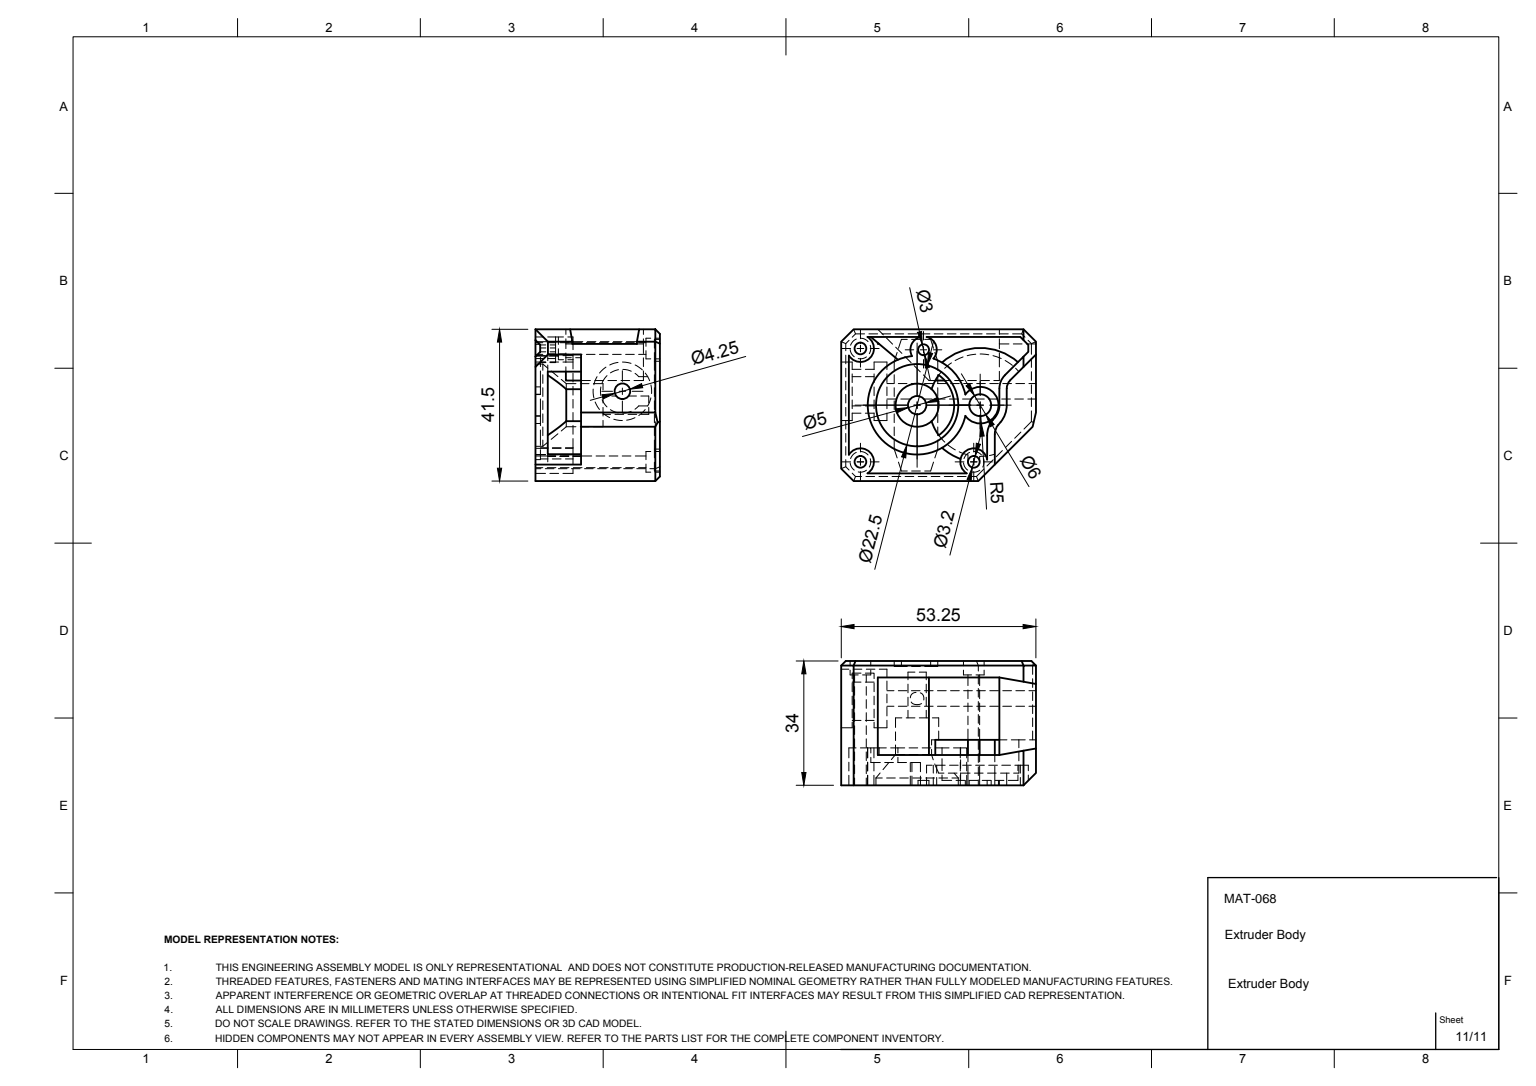
ISO-10303-21;
HEADER;
/* Generated by software containing ST-Developer
 * from STEP Tools, Inc. (www.steptools.com) 
 */

FILE_DESCRIPTION(
/* description */ ('CAx-IF Rec.Pracs.---Representation and Presentation of Product Manufa
cturing Information (PMI)---4.0---2014-10-13'),
/* implementation_level */ '2;1');

FILE_NAME(
/* name */ 'Extruder Body.step',
/* time_stamp */ '2026-10-24T16:53:48-07:00',
/* author */ (''),
/* organization */ (''),
/* preprocessor_version */ 'ST-DEVELOPER v20.2',
/* originating_system */ 'Autodesk Translation Framework v15.17.0.0',
/* authorisation */ '');

FILE_SCHEMA (('AP242_MANAGED_MODEL_BASED_3D_ENGINEERING_MIM_LF { 1 0 10303 442 2 1 4 }'));
ENDSEC;

DATA;
#10=MECHANICAL_DESIGN_GEOMETRIC_PRESENTATION_REPRESENTATION('',(#3498),#107910);
#883=CONICAL_SURFACE('',#50193,0.005875,0.694738276196703);
#2195=B_SPLINE_CURVE_WITH_KNOTS('',3,(#107237,#107238,#107239,#107240,#107241,
#107242,#107243,#107244,#107245,#107246,#107247,#107248,#107249,#107250,
#107251,#107252,#107253,#107254,#107255,#107256,#107257,#107258,#107259,
#107260,#107261,#107262,#107263,#107264,#107265,#107266,#107267,#107268,
#107269,#107270,#107271,#107272,#107273,#107274,#107275,#107276,#107277,
#107278),.UNSPECIFIED.,.T.,.F.,(4,2,2,2,2,2,2,2,2,2,2,2,2,2,2,2,2,2,2,2,
4),(0.,0.0683756752227249,0.13675135044545,0.193430456509981,0.239974549812452,
0.286518643114923,0.333062736417395,0.379606829719866,0.436285935784398,
0.504661611007122,0.573037286229846,0.641412961452571,0.709788636675295,
0.766467742739827,0.813011836042298,0.859555929344769,0.906100022647241,
0.952644115949712,1.00932322201424,1.07769889723697,1.14607457245969),
 .UNSPECIFIED.);
#2196=B_SPLINE_CURVE_WITH_KNOTS('',3,(#107310,#107311,#107312,#107313,#107314,
#107315,#107316,#107317),.UNSPECIFIED.,.F.,.F.,(4,2,2,4),(3.52079202383874,
3.52667424117723,4.17784077952384,4.18520413953086),.UNSPECIFIED.);
#2197=B_SPLINE_CURVE_WITH_KNOTS('',3,(#107322,#107323,#107324,#107325,#107326,
#107327,#107328,#107329),.UNSPECIFIED.,.F.,.F.,(4,2,2,4),(1.56581126613039,
1.57317462613742,2.22434116448402,2.23022338182252),.UNSPECIFIED.);
#3478=SHAPE_REPRESENTATION_RELATIONSHIP('SRR','None',#107956,#3488);
#3488=ADVANCED_BREP_SHAPE_REPRESENTATION('',(#3508),#107909);
#3498=STYLED_ITEM('',(#108007),#3508);
#3508=MANIFOLD_SOLID_BREP('Body1',#45546);
#3523=FACE_BOUND('',#9512,.T.);
#3524=FACE_BOUND('',#9516,.T.);
#3525=FACE_BOUND('',#9542,.T.);
#3526=FACE_BOUND('',#9543,.T.);
#3527=FACE_BOUND('',#9544,.T.);
#3528=FACE_BOUND('',#9545,.T.);
#3529=FACE_BOUND('',#9547,.T.);
#3530=FACE_BOUND('',#9548,.T.);
#3531=FACE_BOUND('',#9549,.T.);
#3532=FACE_BOUND('',#9550,.T.);
#3533=FACE_BOUND('',#9551,.T.);
#3534=FACE_BOUND('',#9552,.T.);
#3535=FACE_BOUND('',#9557,.T.);
#3536=FACE_BOUND('',#9563,.T.);
#3537=FACE_BOUND('',#9573,.T.);
#3538=FACE_BOUND('',#9575,.T.);
#3539=FACE_BOUND('',#9577,.T.);
#3540=FACE_BOUND('',#9607,.T.);
#3541=FACE_BOUND('',#9633,.T.);
#3682=PLANE('',#50239);
#3683=PLANE('',#50245);
#3684=PLANE('',#50248);
#3685=PLANE('',#50249);
#3686=PLANE('',#50250);
#3687=PLANE('',#50251);
#3688=PLANE('',#50263);
#3689=PLANE('',#50264);
#3690=PLANE('',#50265);
#3691=PLANE('',#50266);
#3692=PLANE('',#50276);
#3693=PLANE('',#50277);
#3694=PLANE('',#50278);
#3695=PLANE('',#50279);
#3696=PLANE('',#50280);
#3697=PLANE('',#50281);
#3698=PLANE('',#50282);
#3699=PLANE('',#50283);
#3700=PLANE('',#50284);
#3701=PLANE('',#50285);
#3702=PLANE('',#50286);
#3703=PLANE('',#50287);
#3704=PLANE('',#50288);
#3705=PLANE('',#50289);
#3706=PLANE('',#50290);
#3707=PLANE('',#50291);
#3708=PLANE('',#50292);
#3709=PLANE('',#50293);
#3710=PLANE('',#50294);
#3711=PLANE('',#50295);
#3712=PLANE('',#50296);
#3713=PLANE('',#50299);
#3714=PLANE('',#50302);
#3715=PLANE('',#50305);
#3716=PLANE('',#50308);
#3717=PLANE('',#50309);
#3718=PLANE('',#50310);
#3719=PLANE('',#50311);
#3720=PLANE('',#50314);
#3721=PLANE('',#50317);
#3722=PLANE('',#50318);
#3723=PLANE('',#50319);
#3724=PLANE('',#50321);
#3725=PLANE('',#50323);
#3726=PLANE('',#50325);
#3727=PLANE('',#50326);
#3728=PLANE('',#50329);
#3729=PLANE('',#50330);
#3730=PLANE('',#50331);
#3731=PLANE('',#50332);
#3732=PLANE('',#50333);
#3733=PLANE('',#50334);
#3734=PLANE('',#50335);
#3735=PLANE('',#50336);
#3736=PLANE('',#50337);
#3737=PLANE('',#50338);
#3738=PLANE('',#50339);
#3739=PLANE('',#50340);
#3740=PLANE('',#50341);
#3741=PLANE('',#50342);
#3742=PLANE('',#50345);
#3743=PLANE('',#50346);
#3744=PLANE('',#50349);
#3745=PLANE('',#50350);
#3746=PLANE('',#50351);
#3747=PLANE('',#50352);
#3748=PLANE('',#50353);
#3749=PLANE('',#50354);
#3750=PLANE('',#50355);
#3751=PLANE('',#50356);
#3752=PLANE('',#50357);
#3753=PLANE('',#50358);
#3754=PLANE('',#50359);
#3755=PLANE('',#50363);
#3756=PLANE('',#50364);
#3757=PLANE('',#50365);
#6572=FACE_OUTER_BOUND('',#9510,.T.);
#6573=FACE_OUTER_BOUND('',#9511,.T.);
#6574=FACE_OUTER_BOUND('',#9513,.T.);
#6575=FACE_OUTER_BOUND('',#9514,.T.);
#6576=FACE_OUTER_BOUND('',#9515,.T.);
#6577=FACE_OUTER_BOUND('',#9517,.T.);
#6578=FACE_OUTER_BOUND('',#9518,.T.);
#6579=FACE_OUTER_BOUND('',#9519,.T.);
#6580=FACE_OUTER_BOUND('',#9520,.T.);
#6581=FACE_OUTER_BOUND('',#9521,.T.);
#6582=FACE_OUTER_BOUND('',#9522,.T.);
#6583=FACE_OUTER_BOUND('',#9523,.T.);
#6584=FACE_OUTER_BOUND('',#9524,.T.);
#6585=FACE_OUTER_BOUND('',#9525,.T.);
#6586=FACE_OUTER_BOUND('',#9526,.T.);
#6587=FACE_OUTER_BOUND('',#9527,.T.);
#6588=FACE_OUTER_BOUND('',#9528,.T.);
#6589=FACE_OUTER_BOUND('',#9529,.T.);
#6590=FACE_OUTER_BOUND('',#9530,.T.);
#6591=FACE_OUTER_BOUND('',#9531,.T.);
#6592=FACE_OUTER_BOUND('',#9532,.T.);
#6593=FACE_OUTER_BOUND('',#9533,.T.);
#6594=FACE_OUTER_BOUND('',#9534,.T.);
#6595=FACE_OUTER_BOUND('',#9535,.T.);
#6596=FACE_OUTER_BOUND('',#9536,.T.);
#6597=FACE_OUTER_BOUND('',#9537,.T.);
#6598=FACE_OUTER_BOUND('',#9538,.T.);
#6599=FACE_OUTER_BOUND('',#9539,.T.);
#6600=FACE_OUTER_BOUND('',#9540,.T.);
#6601=FACE_OUTER_BOUND('',#9541,.T.);
#6602=FACE_OUTER_BOUND('',#9546,.T.);
#6603=FACE_OUTER_BOUND('',#9553,.T.);
#6604=FACE_OUTER_BOUND('',#9554,.T.);
#6605=FACE_OUTER_BOUND('',#9555,.T.);
#6606=FACE_OUTER_BOUND('',#9556,.T.);
#6607=FACE_OUTER_BOUND('',#9558,.T.);
#6608=FACE_OUTER_BOUND('',#9559,.T.);
#6609=FACE_OUTER_BOUND('',#9560,.T.);
#6610=FACE_OUTER_BOUND('',#9561,.T.);
#6611=FACE_OUTER_BOUND('',#9562,.T.);
#6612=FACE_OUTER_BOUND('',#9564,.T.);
#6613=FACE_OUTER_BOUND('',#9565,.T.);
#6614=FACE_OUTER_BOUND('',#9566,.T.);
#6615=FACE_OUTER_BOUND('',#9567,.T.);
#6616=FACE_OUTER_BOUND('',#9568,.T.);
#6617=FACE_OUTER_BOUND('',#9569,.T.);
#6618=FACE_OUTER_BOUND('',#9570,.T.);
#6619=FACE_OUTER_BOUND('',#9571,.T.);
#6620=FACE_OUTER_BOUND('',#9572,.T.);
#6621=FACE_OUTER_BOUND('',#9574,.T.);
#6622=FACE_OUTER_BOUND('',#9576,.T.);
#6623=FACE_OUTER_BOUND('',#9578,.T.);
#6624=FACE_OUTER_BOUND('',#9579,.T.);
#6625=FACE_OUTER_BOUND('',#9580,.T.);
#6626=FACE_OUTER_BOUND('',#9581,.T.);
#6627=FACE_OUTER_BOUND('',#9582,.T.);
#6628=FACE_OUTER_BOUND('',#9583,.T.);
#6629=FACE_OUTER_BOUND('',#9584,.T.);
#6630=FACE_OUTER_BOUND('',#9585,.T.);
#6631=FACE_OUTER_BOUND('',#9586,.T.);
#6632=FACE_OUTER_BOUND('',#9587,.T.);
#6633=FACE_OUTER_BOUND('',#9588,.T.);
#6634=FACE_OUTER_BOUND('',#9589,.T.);
#6635=FACE_OUTER_BOUND('',#9590,.T.);
#6636=FACE_OUTER_BOUND('',#9591,.T.);
#6637=FACE_OUTER_BOUND('',#9592,.T.);
#6638=FACE_OUTER_BOUND('',#9593,.T.);
#6639=FACE_OUTER_BOUND('',#9594,.T.);
#6640=FACE_OUTER_BOUND('',#9595,.T.);
#6641=FACE_OUTER_BOUND('',#9596,.T.);
#6642=FACE_OUTER_BOUND('',#9597,.T.);
#6643=FACE_OUTER_BOUND('',#9598,.T.);
#6644=FACE_OUTER_BOUND('',#9599,.T.);
#6645=FACE_OUTER_BOUND('',#9600,.T.);
#6646=FACE_OUTER_BOUND('',#9601,.T.);
#6647=FACE_OUTER_BOUND('',#9602,.T.);
#6648=FACE_OUTER_BOUND('',#9603,.T.);
#6649=FACE_OUTER_BOUND('',#9604,.T.);
#6650=FACE_OUTER_BOUND('',#9605,.T.);
#6651=FACE_OUTER_BOUND('',#9606,.T.);
#6652=FACE_OUTER_BOUND('',#9608,.T.);
#6653=FACE_OUTER_BOUND('',#9609,.T.);
#6654=FACE_OUTER_BOUND('',#9610,.T.);
#6655=FACE_OUTER_BOUND('',#9611,.T.);
#6656=FACE_OUTER_BOUND('',#9612,.T.);
#6657=FACE_OUTER_BOUND('',#9613,.T.);
#6658=FACE_OUTER_BOUND('',#9614,.T.);
#6659=FACE_OUTER_BOUND('',#9615,.T.);
#6660=FACE_OUTER_BOUND('',#9616,.T.);
#6661=FACE_OUTER_BOUND('',#9617,.T.);
#6662=FACE_OUTER_BOUND('',#9618,.T.);
#6663=FACE_OUTER_BOUND('',#9619,.T.);
#6664=FACE_OUTER_BOUND('',#9620,.T.);
#6665=FACE_OUTER_BOUND('',#9621,.T.);
#6666=FACE_OUTER_BOUND('',#9622,.T.);
#6667=FACE_OUTER_BOUND('',#9623,.T.);
#6668=FACE_OUTER_BOUND('',#9624,.T.);
#6669=FACE_OUTER_BOUND('',#9625,.T.);
#6670=FACE_OUTER_BOUND('',#9626,.T.);
#6671=FACE_OUTER_BOUND('',#9627,.T.);
#6672=FACE_OUTER_BOUND('',#9628,.T.);
#6673=FACE_OUTER_BOUND('',#9629,.T.);
#6674=FACE_OUTER_BOUND('',#9630,.T.);
#6675=FACE_OUTER_BOUND('',#9631,.T.);
#6676=FACE_OUTER_BOUND('',#9632,.T.);
#6677=FACE_OUTER_BOUND('',#9634,.T.);
#6678=FACE_OUTER_BOUND('',#9635,.T.);
#6679=FACE_OUTER_BOUND('',#9636,.T.);
#6680=FACE_OUTER_BOUND('',#9637,.T.);
#6681=FACE_OUTER_BOUND('',#9638,.T.);
#9510=EDGE_LOOP('',(#41354,#41355,#41356,#41357,#41358,#41359,#41360,#41361,
#41362,#41363,#41364,#41365));
#9511=EDGE_LOOP('',(#41366,#41367,#41368,#41369));
#9512=EDGE_LOOP('',(#41370));
#9513=EDGE_LOOP('',(#41371,#41372,#41373,#41374));
#9514=EDGE_LOOP('',(#41375,#41376,#41377,#41378));
#9515=EDGE_LOOP('',(#41379,#41380,#41381,#41382));
#9516=EDGE_LOOP('',(#41383));
#9517=EDGE_LOOP('',(#41384,#41385,#41386,#41387,#41388,#41389,#41390,#41391,
#41392));
#9518=EDGE_LOOP('',(#41393,#41394,#41395,#41396));
#9519=EDGE_LOOP('',(#41397,#41398,#41399,#41400));
#9520=EDGE_LOOP('',(#41401,#41402,#41403,#41404));
#9521=EDGE_LOOP('',(#41405,#41406,#41407,#41408,#41409,#41410));
#9522=EDGE_LOOP('',(#41411,#41412,#41413,#41414));
#9523=EDGE_LOOP('',(#41415,#41416,#41417,#41418));
#9524=EDGE_LOOP('',(#41419,#41420,#41421,#41422));
#9525=EDGE_LOOP('',(#41423,#41424,#41425,#41426));
#9526=EDGE_LOOP('',(#41427,#41428,#41429,#41430,#41431,#41432,#41433,#41434,
#41435,#41436));
#9527=EDGE_LOOP('',(#41437,#41438,#41439,#41440));
#9528=EDGE_LOOP('',(#41441,#41442,#41443,#41444,#41445,#41446,#41447,#41448));
#9529=EDGE_LOOP('',(#41449,#41450,#41451,#41452,#41453,#41454,#41455,#41456));
#9530=EDGE_LOOP('',(#41457,#41458,#41459,#41460));
#9531=EDGE_LOOP('',(#41461,#41462,#41463,#41464,#41465,#41466,#41467,#41468,
#41469));
#9532=EDGE_LOOP('',(#41470,#41471,#41472,#41473,#41474,#41475,#41476,#41477,
#41478,#41479,#41480,#41481,#41482,#41483,#41484));
#9533=EDGE_LOOP('',(#41485,#41486,#41487,#41488,#41489,#41490));
#9534=EDGE_LOOP('',(#41491,#41492,#41493,#41494,#41495));
#9535=EDGE_LOOP('',(#41496,#41497,#41498,#41499));
#9536=EDGE_LOOP('',(#41500,#41501,#41502,#41503,#41504,#41505,#41506,#41507,
#41508,#41509,#41510,#41511,#41512));
#9537=EDGE_LOOP('',(#41513,#41514,#41515,#41516,#41517,#41518));
#9538=EDGE_LOOP('',(#41519,#41520,#41521,#41522,#41523));
#9539=EDGE_LOOP('',(#41524,#41525,#41526,#41527));
#9540=EDGE_LOOP('',(#41528,#41529,#41530,#41531,#41532,#41533));
#9541=EDGE_LOOP('',(#41534,#41535,#41536,#41537,#41538,#41539,#41540,#41541));
#9542=EDGE_LOOP('',(#41542,#41543,#41544,#41545,#41546,#41547,#41548,#41549));
#9543=EDGE_LOOP('',(#41550));
#9544=EDGE_LOOP('',(#41551));
#9545=EDGE_LOOP('',(#41552));
#9546=EDGE_LOOP('',(#41553,#41554,#41555,#41556,#41557,#41558,#41559,#41560,
#41561,#41562,#41563,#41564,#41565,#41566,#41567,#41568,#41569,#41570,#41571,
#41572,#41573,#41574,#41575,#41576,#41577,#41578,#41579,#41580,#41581,#41582,
#41583,#41584,#41585,#41586,#41587));
#9547=EDGE_LOOP('',(#41588));
#9548=EDGE_LOOP('',(#41589));
#9549=EDGE_LOOP('',(#41590));
#9550=EDGE_LOOP('',(#41591));
#9551=EDGE_LOOP('',(#41592));
#9552=EDGE_LOOP('',(#41593));
#9553=EDGE_LOOP('',(#41594,#41595,#41596,#41597));
#9554=EDGE_LOOP('',(#41598,#41599,#41600,#41601,#41602,#41603,#41604,#41605,
#41606,#41607));
#9555=EDGE_LOOP('',(#41608,#41609,#41610,#41611));
#9556=EDGE_LOOP('',(#41612,#41613,#41614,#41615,#41616,#41617,#41618,#41619,
#41620,#41621));
#9557=EDGE_LOOP('',(#41622));
#9558=EDGE_LOOP('',(#41623,#41624,#41625,#41626,#41627));
#9559=EDGE_LOOP('',(#41628,#41629,#41630,#41631,#41632,#41633));
#9560=EDGE_LOOP('',(#41634,#41635,#41636,#41637));
#9561=EDGE_LOOP('',(#41638,#41639,#41640,#41641));
#9562=EDGE_LOOP('',(#41642,#41643,#41644,#41645));
#9563=EDGE_LOOP('',(#41646));
#9564=EDGE_LOOP('',(#41647,#41648,#41649,#41650));
#9565=EDGE_LOOP('',(#41651,#41652,#41653,#41654));
#9566=EDGE_LOOP('',(#41655,#41656,#41657,#41658));
#9567=EDGE_LOOP('',(#41659,#41660,#41661,#41662));
#9568=EDGE_LOOP('',(#41663,#41664,#41665,#41666));
#9569=EDGE_LOOP('',(#41667,#41668,#41669,#41670,#41671));
#9570=EDGE_LOOP('',(#41672,#41673,#41674,#41675));
#9571=EDGE_LOOP('',(#41676,#41677,#41678,#41679,#41680));
#9572=EDGE_LOOP('',(#41681));
#9573=EDGE_LOOP('',(#41682));
#9574=EDGE_LOOP('',(#41683));
#9575=EDGE_LOOP('',(#41684));
#9576=EDGE_LOOP('',(#41685));
#9577=EDGE_LOOP('',(#41686));
#9578=EDGE_LOOP('',(#41687,#41688,#41689,#41690,#41691,#41692,#41693));
#9579=EDGE_LOOP('',(#41694,#41695,#41696,#41697));
#9580=EDGE_LOOP('',(#41698,#41699,#41700,#41701));
#9581=EDGE_LOOP('',(#41702,#41703,#41704,#41705));
#9582=EDGE_LOOP('',(#41706,#41707,#41708,#41709));
#9583=EDGE_LOOP('',(#41710,#41711,#41712,#41713));
#9584=EDGE_LOOP('',(#41714,#41715,#41716,#41717,#41718,#41719));
#9585=EDGE_LOOP('',(#41720,#41721,#41722,#41723));
#9586=EDGE_LOOP('',(#41724,#41725,#41726,#41727,#41728,#41729,#41730,#41731,
#41732,#41733,#41734,#41735,#41736,#41737,#41738));
#9587=EDGE_LOOP('',(#41739,#41740,#41741,#41742));
#9588=EDGE_LOOP('',(#41743,#41744,#41745,#41746));
#9589=EDGE_LOOP('',(#41747,#41748,#41749,#41750));
#9590=EDGE_LOOP('',(#41751,#41752,#41753,#41754));
#9591=EDGE_LOOP('',(#41755,#41756,#41757,#41758));
#9592=EDGE_LOOP('',(#41759,#41760,#41761,#41762));
#9593=EDGE_LOOP('',(#41763,#41764,#41765,#41766,#41767));
#9594=EDGE_LOOP('',(#41768,#41769,#41770,#41771));
#9595=EDGE_LOOP('',(#41772,#41773,#41774,#41775,#41776,#41777,#41778));
#9596=EDGE_LOOP('',(#41779,#41780,#41781,#41782));
#9597=EDGE_LOOP('',(#41783,#41784,#41785,#41786));
#9598=EDGE_LOOP('',(#41787,#41788,#41789,#41790));
#9599=EDGE_LOOP('',(#41791,#41792,#41793,#41794));
#9600=EDGE_LOOP('',(#41795,#41796,#41797,#41798));
#9601=EDGE_LOOP('',(#41799,#41800,#41801,#41802));
#9602=EDGE_LOOP('',(#41803,#41804,#41805,#41806,#41807,#41808,#41809,#41810));
#9603=EDGE_LOOP('',(#41811,#41812,#41813,#41814));
#9604=EDGE_LOOP('',(#41815));
#9605=EDGE_LOOP('',(#41816,#41817,#41818,#41819));
#9606=EDGE_LOOP('',(#41820));
#9607=EDGE_LOOP('',(#41821));
#9608=EDGE_LOOP('',(#41822));
#9609=EDGE_LOOP('',(#41823));
#9610=EDGE_LOOP('',(#41824,#41825,#41826,#41827));
#9611=EDGE_LOOP('',(#41828,#41829,#41830,#41831));
#9612=EDGE_LOOP('',(#41832,#41833,#41834,#41835));
#9613=EDGE_LOOP('',(#41836,#41837,#41838,#41839));
#9614=EDGE_LOOP('',(#41840,#41841,#41842,#41843));
#9615=EDGE_LOOP('',(#41844,#41845,#41846,#41847));
#9616=EDGE_LOOP('',(#41848,#41849,#41850,#41851));
#9617=EDGE_LOOP('',(#41852,#41853,#41854,#41855));
#9618=EDGE_LOOP('',(#41856,#41857,#41858,#41859,#41860,#41861,#41862,#41863));
#9619=EDGE_LOOP('',(#41864,#41865,#41866,#41867));
#9620=EDGE_LOOP('',(#41868,#41869,#41870,#41871,#41872,#41873,#41874));
#9621=EDGE_LOOP('',(#41875,#41876,#41877,#41878,#41879,#41880,#41881,#41882));
#9622=EDGE_LOOP('',(#41883,#41884,#41885,#41886));
#9623=EDGE_LOOP('',(#41887,#41888,#41889,#41890,#41891,#41892,#41893,#41894,
#41895,#41896,#41897,#41898));
#9624=EDGE_LOOP('',(#41899,#41900,#41901,#41902,#41903));
#9625=EDGE_LOOP('',(#41904,#41905,#41906,#41907,#41908));
#9626=EDGE_LOOP('',(#41909,#41910,#41911,#41912));
#9627=EDGE_LOOP('',(#41913,#41914,#41915));
#9628=EDGE_LOOP('',(#41916,#41917,#41918,#41919));
#9629=EDGE_LOOP('',(#41920,#41921,#41922,#41923));
#9630=EDGE_LOOP('',(#41924,#41925,#41926,#41927,#41928,#41929));
#9631=EDGE_LOOP('',(#41930,#41931,#41932,#41933,#41934,#41935));
#9632=EDGE_LOOP('',(#41936));
#9633=EDGE_LOOP('',(#41937));
#9634=EDGE_LOOP('',(#41938,#41939,#41940,#41941,#41942));
#9635=EDGE_LOOP('',(#41943,#41944,#41945,#41946));
#9636=EDGE_LOOP('',(#41947,#41948,#41949,#41950,#41951));
#9637=EDGE_LOOP('',(#41952,#41953,#41954,#41955));
#9638=EDGE_LOOP('',(#41956,#41957,#41958,#41959));
#11405=LINE('',#107215,#13389);
#11406=LINE('',#107219,#13390);
#11407=LINE('',#107223,#13391);
#11408=LINE('',#107228,#13392);
#11409=LINE('',#107234,#13393);
#11410=LINE('',#107283,#13394);
#11411=LINE('',#107290,#13395);
#11412=LINE('',#107293,#13396);
#11413=LINE('',#107298,#13397);
#11414=LINE('',#107305,#13398);
#11415=LINE('',#107332,#13399);
#11416=LINE('',#107338,#13400);
#11417=LINE('',#107345,#13401);
#11418=LINE('',#107348,#13402);
#11419=LINE('',#107354,#13403);
#11420=LINE('',#107358,#13404);
#11421=LINE('',#107361,#13405);
#11422=LINE('',#107366,#13406);
#11423=LINE('',#107372,#13407);
#11424=LINE('',#107378,#13408);
#11425=LINE('',#107384,#13409);
#11426=LINE('',#107390,#13410);
#11427=LINE('',#107394,#13411);
#11428=LINE('',#107398,#13412);
#11429=LINE('',#107400,#13413);
#11430=LINE('',#107405,#13414);
#11431=LINE('',#107409,#13415);
#11432=LINE('',#107412,#13416);
#11433=LINE('',#107415,#13417);
#11434=LINE('',#107421,#13418);
#11435=LINE('',#107426,#13419);
#11436=LINE('',#107429,#13420);
#11437=LINE('',#107433,#13421);
#11438=LINE('',#107435,#13422);
#11439=LINE('',#107437,#13423);
#11440=LINE('',#107438,#13424);
#11441=LINE('',#107442,#13425);
#11442=LINE('',#107446,#13426);
#11443=LINE('',#107450,#13427);
#11444=LINE('',#107455,#13428);
#11445=LINE('',#107458,#13429);
#11446=LINE('',#107460,#13430);
#11447=LINE('',#107464,#13431);
#11448=LINE('',#107466,#13432);
#11449=LINE('',#107468,#13433);
#11450=LINE('',#107470,#13434);
#11451=LINE('',#107471,#13435);
#11452=LINE('',#107472,#13436);
#11453=LINE('',#107476,#13437);
#11454=LINE('',#107478,#13438);
#11455=LINE('',#107479,#13439);
#11456=LINE('',#107480,#13440);
#11457=LINE('',#107481,#13441);
#11458=LINE('',#107485,#13442);
#11459=LINE('',#107487,#13443);
#11460=LINE('',#107488,#13444);
#11461=LINE('',#107490,#13445);
#11462=LINE('',#107491,#13446);
#11463=LINE('',#107495,#13447);
#11464=LINE('',#107497,#13448);
#11465=LINE('',#107499,#13449);
#11466=LINE('',#107500,#13450);
#11467=LINE('',#107504,#13451);
#11468=LINE('',#107508,#13452);
#11469=LINE('',#107512,#13453);
#11470=LINE('',#107516,#13454);
#11471=LINE('',#107522,#13455);
#11472=LINE('',#107528,#13456);
#11473=LINE('',#107531,#13457);
#11474=LINE('',#107533,#13458);
#11475=LINE('',#107534,#13459);
#11476=LINE('',#107538,#13460);
#11477=LINE('',#107540,#13461);
#11478=LINE('',#107542,#13462);
#11479=LINE('',#107544,#13463);
#11480=LINE('',#107546,#13464);
#11481=LINE('',#107547,#13465);
#11482=LINE('',#107551,#13466);
#11483=LINE('',#107553,#13467);
#11484=LINE('',#107555,#13468);
#11485=LINE('',#107557,#13469);
#11486=LINE('',#107559,#13470);
#11487=LINE('',#107561,#13471);
#11488=LINE('',#107563,#13472);
#11489=LINE('',#107564,#13473);
#11490=LINE('',#107567,#13474);
#11491=LINE('',#107569,#13475);
#11492=LINE('',#107571,#13476);
#11493=LINE('',#107573,#13477);
#11494=LINE('',#107575,#13478);
#11495=LINE('',#107577,#13479);
#11496=LINE('',#107579,#13480);
#11497=LINE('',#107580,#13481);
#11498=LINE('',#107583,#13482);
#11499=LINE('',#107585,#13483);
#11500=LINE('',#107587,#13484);
#11501=LINE('',#107589,#13485);
#11502=LINE('',#107591,#13486);
#11503=LINE('',#107593,#13487);
#11504=LINE('',#107595,#13488);
#11505=LINE('',#107597,#13489);
#11506=LINE('',#107599,#13490);
#11507=LINE('',#107603,#13491);
#11508=LINE('',#107607,#13492);
#11509=LINE('',#107611,#13493);
#11510=LINE('',#107613,#13494);
#11511=LINE('',#107615,#13495);
#11512=LINE('',#107619,#13496);
#11513=LINE('',#107623,#13497);
#11514=LINE('',#107626,#13498);
#11515=LINE('',#107628,#13499);
#11516=LINE('',#107632,#13500);
#11517=LINE('',#107637,#13501);
#11518=LINE('',#107639,#13502);
#11519=LINE('',#107640,#13503);
#11520=LINE('',#107642,#13504);
#11521=LINE('',#107643,#13505);
#11522=LINE('',#107645,#13506);
#11523=LINE('',#107646,#13507);
#11524=LINE('',#107647,#13508);
#11525=LINE('',#107651,#13509);
#11526=LINE('',#107652,#13510);
#11527=LINE('',#107653,#13511);
#11528=LINE('',#107655,#13512);
#11529=LINE('',#107656,#13513);
#11530=LINE('',#107658,#13514);
#11531=LINE('',#107659,#13515);
#11532=LINE('',#107661,#13516);
#11533=LINE('',#107662,#13517);
#11534=LINE('',#107665,#13518);
#11535=LINE('',#107667,#13519);
#11536=LINE('',#107668,#13520);
#11537=LINE('',#107670,#13521);
#11538=LINE('',#107672,#13522);
#11539=LINE('',#107673,#13523);
#11540=LINE('',#107676,#13524);
#11541=LINE('',#107677,#13525);
#11542=LINE('',#107680,#13526);
#11543=LINE('',#107681,#13527);
#11544=LINE('',#107683,#13528);
#11545=LINE('',#107685,#13529);
#11546=LINE('',#107686,#13530);
#11547=LINE('',#107688,#13531);
#11548=LINE('',#107690,#13532);
#11549=LINE('',#107692,#13533);
#11550=LINE('',#107694,#13534);
#11551=LINE('',#107696,#13535);
#11552=LINE('',#107698,#13536);
#11553=LINE('',#107704,#13537);
#11554=LINE('',#107706,#13538);
#11555=LINE('',#107707,#13539);
#11556=LINE('',#107710,#13540);
#11557=LINE('',#107714,#13541);
#11558=LINE('',#107715,#13542);
#11559=LINE('',#107718,#13543);
#11560=LINE('',#107722,#13544);
#11561=LINE('',#107723,#13545);
#11562=LINE('',#107726,#13546);
#11563=LINE('',#107730,#13547);
#11564=LINE('',#107731,#13548);
#11565=LINE('',#107734,#13549);
#11566=LINE('',#107737,#13550);
#11567=LINE('',#107738,#13551);
#11568=LINE('',#107743,#13552);
#11569=LINE('',#107744,#13553);
#11570=LINE('',#107748,#13554);
#11571=LINE('',#107751,#13555);
#11572=LINE('',#107752,#13556);
#11573=LINE('',#107758,#13557);
#11574=LINE('',#107759,#13558);
#11575=LINE('',#107760,#13559);
#11576=LINE('',#107764,#13560);
#11577=LINE('',#107765,#13561);
#11578=LINE('',#107766,#13562);
#11579=LINE('',#107768,#13563);
#11580=LINE('',#107770,#13564);
#11581=LINE('',#107771,#13565);
#11582=LINE('',#107772,#13566);
#11583=LINE('',#107774,#13567);
#11584=LINE('',#107776,#13568);
#11585=LINE('',#107778,#13569);
#11586=LINE('',#107780,#13570);
#11587=LINE('',#107782,#13571);
#11588=LINE('',#107789,#13572);
#11589=LINE('',#107795,#13573);
#11590=LINE('',#107797,#13574);
#11591=LINE('',#107798,#13575);
#11592=LINE('',#107801,#13576);
#11593=LINE('',#107802,#13577);
#11594=LINE('',#107805,#13578);
#11595=LINE('',#107806,#13579);
#11596=LINE('',#107809,#13580);
#11597=LINE('',#107810,#13581);
#11598=LINE('',#107813,#13582);
#11599=LINE('',#107814,#13583);
#11600=LINE('',#107817,#13584);
#11601=LINE('',#107818,#13585);
#11602=LINE('',#107821,#13586);
#11603=LINE('',#107822,#13587);
#11604=LINE('',#107824,#13588);
#11605=LINE('',#107831,#13589);
#11606=LINE('',#107833,#13590);
#11607=LINE('',#107835,#13591);
#11608=LINE('',#107837,#13592);
#11609=LINE('',#107838,#13593);
#11610=LINE('',#107843,#13594);
#11611=LINE('',#107844,#13595);
#11612=LINE('',#107848,#13596);
#11613=LINE('',#107851,#13597);
#11614=LINE('',#107852,#13598);
#11615=LINE('',#107854,#13599);
#11616=LINE('',#107857,#13600);
#11617=LINE('',#107864,#13601);
#11618=LINE('',#107865,#13602);
#11619=LINE('',#107870,#13603);
#11620=LINE('',#107871,#13604);
#11621=LINE('',#107873,#13605);
#11622=LINE('',#107874,#13606);
#13389=VECTOR('',#61178,0.008);
#13390=VECTOR('',#61181,1.);
#13391=VECTOR('',#61184,0.008);
#13392=VECTOR('',#61189,1.);
#13393=VECTOR('',#61196,0.002125);
#13394=VECTOR('',#61203,0.003);
#13395=VECTOR('',#61210,1.);
#13396=VECTOR('',#61213,1.);
#13397=VECTOR('',#61218,0.0025);
#13398=VECTOR('',#61225,0.005875);
#13399=VECTOR('',#61236,0.01125);
#13400=VECTOR('',#61243,0.0015);
#13401=VECTOR('',#61250,1.);
#13402=VECTOR('',#61253,1.);
#13403=VECTOR('',#61258,1.);
#13404=VECTOR('',#61261,1.);
#13405=VECTOR('',#61264,1.);
#13406=VECTOR('',#61269,0.002825);
#13407=VECTOR('',#61276,0.002825);
#13408=VECTOR('',#61283,0.002825);
#13409=VECTOR('',#61290,0.0016);
#13410=VECTOR('',#61297,0.0016);
#13411=VECTOR('',#61300,1.);
#13412=VECTOR('',#61303,0.0016);
#13413=VECTOR('',#61306,1.);
#13414=VECTOR('',#61311,0.0016);
#13415=VECTOR('',#61316,0.0059);
#13416=VECTOR('',#61319,1.);
#13417=VECTOR('',#61322,1.);
#13418=VECTOR('',#61327,1.);
#13419=VECTOR('',#61332,1.);
#13420=VECTOR('',#61335,1.);
#13421=VECTOR('',#61338,1.);
#13422=VECTOR('',#61339,1.);
#13423=VECTOR('',#61340,1.);
#13424=VECTOR('',#61341,1.);
#13425=VECTOR('',#61344,1.);
#13426=VECTOR('',#61347,1.);
#13427=VECTOR('',#61350,1.);
#13428=VECTOR('',#61357,1.);
#13429=VECTOR('',#61360,1.);
#13430=VECTOR('',#61361,1.);
#13431=VECTOR('',#61364,1.);
#13432=VECTOR('',#61365,1.);
#13433=VECTOR('',#61366,1.);
#13434=VECTOR('',#61367,1.);
#13435=VECTOR('',#61368,1.);
#13436=VECTOR('',#61369,1.);
#13437=VECTOR('',#61372,1.);
#13438=VECTOR('',#61373,1.);
#13439=VECTOR('',#61374,1.);
#13440=VECTOR('',#61375,1.);
#13441=VECTOR('',#61376,1.);
#13442=VECTOR('',#61379,1.);
#13443=VECTOR('',#61380,1.);
#13444=VECTOR('',#61381,1.);
#13445=VECTOR('',#61382,1.);
#13446=VECTOR('',#61383,1.);
#13447=VECTOR('',#61386,1.);
#13448=VECTOR('',#61387,1.);
#13449=VECTOR('',#61388,1.);
#13450=VECTOR('',#61389,1.);
#13451=VECTOR('',#61394,1.);
#13452=VECTOR('',#61397,1.);
#13453=VECTOR('',#61400,1.);
#13454=VECTOR('',#61403,1.);
#13455=VECTOR('',#61410,1.);
#13456=VECTOR('',#61419,1.);
#13457=VECTOR('',#61422,1.);
#13458=VECTOR('',#61423,1.);
#13459=VECTOR('',#61424,1.);
#13460=VECTOR('',#61427,1.);
#13461=VECTOR('',#61428,1.);
#13462=VECTOR('',#61429,1.);
#13463=VECTOR('',#61430,1.);
#13464=VECTOR('',#61431,1.);
#13465=VECTOR('',#61432,1.);
#13466=VECTOR('',#61435,1.);
#13467=VECTOR('',#61436,1.);
#13468=VECTOR('',#61437,1.);
#13469=VECTOR('',#61438,1.);
#13470=VECTOR('',#61439,1.);
#13471=VECTOR('',#61440,1.);
#13472=VECTOR('',#61441,1.);
#13473=VECTOR('',#61442,1.);
#13474=VECTOR('',#61443,1.);
#13475=VECTOR('',#61444,1.);
#13476=VECTOR('',#61445,1.);
#13477=VECTOR('',#61446,1.);
#13478=VECTOR('',#61447,1.);
#13479=VECTOR('',#61448,1.);
#13480=VECTOR('',#61449,1.);
#13481=VECTOR('',#61450,1.);
#13482=VECTOR('',#61453,1.);
#13483=VECTOR('',#61454,1.);
#13484=VECTOR('',#61455,1.);
#13485=VECTOR('',#61456,1.);
#13486=VECTOR('',#61457,1.);
#13487=VECTOR('',#61458,1.);
#13488=VECTOR('',#61459,1.);
#13489=VECTOR('',#61460,1.);
#13490=VECTOR('',#61461,1.);
#13491=VECTOR('',#61464,1.);
#13492=VECTOR('',#61467,1.);
#13493=VECTOR('',#61470,1.);
#13494=VECTOR('',#61471,1.);
#13495=VECTOR('',#61472,1.);
#13496=VECTOR('',#61475,1.);
#13497=VECTOR('',#61478,1.);
#13498=VECTOR('',#61481,1.);
#13499=VECTOR('',#61482,1.);
#13500=VECTOR('',#61485,1.);
#13501=VECTOR('',#61492,1.);
#13502=VECTOR('',#61493,1.);
#13503=VECTOR('',#61494,1.);
#13504=VECTOR('',#61497,1.);
#13505=VECTOR('',#61498,1.);
#13506=VECTOR('',#61499,1.);
#13507=VECTOR('',#61500,1.);
#13508=VECTOR('',#61501,1.);
#13509=VECTOR('',#61504,1.);
#13510=VECTOR('',#61505,1.);
#13511=VECTOR('',#61506,1.);
#13512=VECTOR('',#61509,1.);
#13513=VECTOR('',#61510,1.);
#13514=VECTOR('',#61511,1.);
#13515=VECTOR('',#61512,1.);
#13516=VECTOR('',#61513,1.);
#13517=VECTOR('',#61514,1.);
#13518=VECTOR('',#61517,1.);
#13519=VECTOR('',#61518,1.);
#13520=VECTOR('',#61519,1.);
#13521=VECTOR('',#61522,1.);
#13522=VECTOR('',#61523,1.);
#13523=VECTOR('',#61524,1.);
#13524=VECTOR('',#61527,1.);
#13525=VECTOR('',#61528,1.);
#13526=VECTOR('',#61531,1.);
#13527=VECTOR('',#61532,1.);
#13528=VECTOR('',#61535,1.);
#13529=VECTOR('',#61538,1.);
#13530=VECTOR('',#61539,1.);
#13531=VECTOR('',#61542,1.);
#13532=VECTOR('',#61545,1.);
#13533=VECTOR('',#61548,1.);
#13534=VECTOR('',#61551,1.);
#13535=VECTOR('',#61554,1.);
#13536=VECTOR('',#61557,1.);
#13537=VECTOR('',#61568,1.);
#13538=VECTOR('',#61569,1.);
#13539=VECTOR('',#61570,1.);
#13540=VECTOR('',#61573,1.);
#13541=VECTOR('',#61578,1.);
#13542=VECTOR('',#61579,1.);
#13543=VECTOR('',#61582,1.);
#13544=VECTOR('',#61587,1.);
#13545=VECTOR('',#61588,1.);
#13546=VECTOR('',#61591,1.);
#13547=VECTOR('',#61596,1.);
#13548=VECTOR('',#61597,1.);
#13549=VECTOR('',#61600,1.);
#13550=VECTOR('',#61605,1.);
#13551=VECTOR('',#61606,1.);
#13552=VECTOR('',#61613,1.);
#13553=VECTOR('',#61614,1.);
#13554=VECTOR('',#61619,1.);
#13555=VECTOR('',#61622,1.);
#13556=VECTOR('',#61623,1.);
#13557=VECTOR('',#61630,1.);
#13558=VECTOR('',#61631,1.);
#13559=VECTOR('',#61632,1.);
#13560=VECTOR('',#61635,1.);
#13561=VECTOR('',#61636,1.);
#13562=VECTOR('',#61637,1.);
#13563=VECTOR('',#61640,1.);
#13564=VECTOR('',#61641,1.);
#13565=VECTOR('',#61642,1.);
#13566=VECTOR('',#61643,1.);
#13567=VECTOR('',#61646,1.);
#13568=VECTOR('',#61649,1.);
#13569=VECTOR('',#61652,1.);
#13570=VECTOR('',#61655,1.);
#13571=VECTOR('',#61658,1.);
#13572=VECTOR('',#61671,1.);
#13573=VECTOR('',#61680,1.);
#13574=VECTOR('',#61681,1.);
#13575=VECTOR('',#61682,1.);
#13576=VECTOR('',#61685,1.);
#13577=VECTOR('',#61686,1.);
#13578=VECTOR('',#61689,1.);
#13579=VECTOR('',#61690,1.);
#13580=VECTOR('',#61693,1.);
#13581=VECTOR('',#61694,1.);
#13582=VECTOR('',#61697,1.);
#13583=VECTOR('',#61698,1.);
#13584=VECTOR('',#61701,1.);
#13585=VECTOR('',#61702,1.);
#13586=VECTOR('',#61705,1.);
#13587=VECTOR('',#61706,1.);
#13588=VECTOR('',#61709,1.);
#13589=VECTOR('',#61720,1.);
#13590=VECTOR('',#61721,1.);
#13591=VECTOR('',#61722,1.);
#13592=VECTOR('',#61723,1.);
#13593=VECTOR('',#61724,1.);
#13594=VECTOR('',#61731,1.);
#13595=VECTOR('',#61732,1.);
#13596=VECTOR('',#61739,1.);
#13597=VECTOR('',#61742,1.);
#13598=VECTOR('',#61743,1.);
#13599=VECTOR('',#61746,1.);
#13600=VECTOR('',#61751,1.);
#13601=VECTOR('',#61760,1.);
#13602=VECTOR('',#61761,1.);
#13603=VECTOR('',#61766,1.);
#13604=VECTOR('',#61767,1.);
#13605=VECTOR('',#61770,1.);
#13606=VECTOR('',#61771,1.);
#17097=CIRCLE('',#50175,0.00800000000000999);
#17098=CIRCLE('',#50176,0.00800000000000999);
#17099=CIRCLE('',#50177,0.00800000000000999);
#17100=CIRCLE('',#50178,0.00800000000000999);
#17101=CIRCLE('',#50179,0.00800000000000999);
#17102=CIRCLE('',#50180,0.00800000000000999);
#17103=CIRCLE('',#50182,0.00212500000001);
#17104=CIRCLE('',#50183,0.00212500000001);
#17105=CIRCLE('',#50185,0.00300000000001);
#17106=CIRCLE('',#50186,0.00300000000001);
#17107=CIRCLE('',#50188,0.00500000000001);
#17108=CIRCLE('',#50189,0.00500000000001);
#17109=CIRCLE('',#50191,0.00250000000001);
#17110=CIRCLE('',#50192,0.00250000000001);
#17111=CIRCLE('',#50194,0.01012500000001);
#17112=CIRCLE('',#50195,0.01125000000001);
#17113=CIRCLE('',#50196,0.01012500000001);
#17114=CIRCLE('',#50197,0.00590000000001);
#17115=CIRCLE('',#50198,0.00590000000001);
#17116=CIRCLE('',#50200,0.01125000000001);
#17117=CIRCLE('',#50202,0.00150000000001);
#17118=CIRCLE('',#50203,0.00150000000001);
#17119=CIRCLE('',#50205,0.00360000000001);
#17120=CIRCLE('',#50206,0.00360000000001);
#17121=CIRCLE('',#50208,0.00370000000001);
#17122=CIRCLE('',#50209,0.00370000000001);
#17123=CIRCLE('',#50210,0.00370000000001);
#17124=CIRCLE('',#50212,0.00282500000001);
#17125=CIRCLE('',#50213,0.00282500000001);
#17126=CIRCLE('',#50215,0.00282500000001);
#17127=CIRCLE('',#50216,0.00282500000001);
#17128=CIRCLE('',#50218,0.00282500000001);
#17129=CIRCLE('',#50219,0.00282500000001);
#17130=CIRCLE('',#50221,0.00160000000001);
#17131=CIRCLE('',#50222,0.00160000000001);
#17132=CIRCLE('',#50224,0.00160000000001);
#17133=CIRCLE('',#50225,0.00160000000001);
#17134=CIRCLE('',#50226,0.00160000000001);
#17135=CIRCLE('',#50227,0.00160000000001);
#17136=CIRCLE('',#50229,0.00160000000001);
#17137=CIRCLE('',#50230,0.00160000000001);
#17138=CIRCLE('',#50232,0.00590000000001);
#17139=CIRCLE('',#50233,0.00590000000001);
#17140=CIRCLE('',#50235,0.01350000000001);
#17141=CIRCLE('',#50236,0.01350000000001);
#17142=CIRCLE('',#50237,0.01350000000001);
#17143=CIRCLE('',#50238,0.01350000000001);
#17144=CIRCLE('',#50241,0.01400000000001);
#17145=CIRCLE('',#50242,0.01400000000001);
#17146=CIRCLE('',#50243,0.01400000000001);
#17147=CIRCLE('',#50244,0.01400000000001);
#17148=CIRCLE('',#50246,0.01400000000001);
#17149=CIRCLE('',#50247,0.01400000000001);
#17150=CIRCLE('',#50252,0.01565000000001);
#17151=CIRCLE('',#50253,0.00650498845855181);
#17152=CIRCLE('',#50254,0.00525000000001);
#17153=CIRCLE('',#50255,0.00500000000001);
#17154=CIRCLE('',#50256,0.01565000000001);
#17155=CIRCLE('',#50257,0.01350000000001);
#17156=CIRCLE('',#50259,0.01350000000001);
#17157=CIRCLE('',#50260,0.01350000000001);
#17158=CIRCLE('',#50262,0.01400000000001);
#17159=CIRCLE('',#50267,0.00400000000001);
#17160=CIRCLE('',#50268,0.00725000000001);
#17161=CIRCLE('',#50269,0.00300000000001001);
#17162=CIRCLE('',#50270,0.00500000000001);
#17163=CIRCLE('',#50271,0.00525000000001);
#17164=CIRCLE('',#50272,0.00650498845855181);
#17165=CIRCLE('',#50273,0.00370000000001);
#17166=CIRCLE('',#50274,0.00370000000001);
#17167=CIRCLE('',#50275,0.00360000000001);
#17168=CIRCLE('',#50298,0.00300000000001001);
#17169=CIRCLE('',#50301,0.00725000000001);
#17170=CIRCLE('',#50304,0.00400000000001);
#17171=CIRCLE('',#50307,0.01400000000001);
#17172=CIRCLE('',#50313,0.00370000000001);
#17173=CIRCLE('',#50316,0.00370000000001);
#17174=CIRCLE('',#50328,0.00360000000001);
#17175=CIRCLE('',#50344,0.01565000000001);
#17176=CIRCLE('',#50348,0.01565000000001);
#17177=CIRCLE('',#50360,0.00600000000001);
#17178=CIRCLE('',#50362,0.00600000000001);
#21005=VERTEX_POINT('',#107212);
#21006=VERTEX_POINT('',#107214);
#21007=VERTEX_POINT('',#107216);
#21008=VERTEX_POINT('',#107218);
#21009=VERTEX_POINT('',#107220);
#21010=VERTEX_POINT('',#107222);
#21011=VERTEX_POINT('',#107225);
#21012=VERTEX_POINT('',#107227);
#21013=VERTEX_POINT('',#107231);
#21014=VERTEX_POINT('',#107233);
#21015=VERTEX_POINT('',#107236);
#21016=VERTEX_POINT('',#107280);
#21017=VERTEX_POINT('',#107282);
#21018=VERTEX_POINT('',#107286);
#21019=VERTEX_POINT('',#107287);
#21020=VERTEX_POINT('',#107289);
#21021=VERTEX_POINT('',#107291);
#21022=VERTEX_POINT('',#107295);
#21023=VERTEX_POINT('',#107297);
#21024=VERTEX_POINT('',#107301);
#21025=VERTEX_POINT('',#107302);
#21026=VERTEX_POINT('',#107304);
#21027=VERTEX_POINT('',#107307);
#21028=VERTEX_POINT('',#107309);
#21029=VERTEX_POINT('',#107318);
#21030=VERTEX_POINT('',#107320);
#21031=VERTEX_POINT('',#107331);
#21032=VERTEX_POINT('',#107335);
#21033=VERTEX_POINT('',#107337);
#21034=VERTEX_POINT('',#107341);
#21035=VERTEX_POINT('',#107342);
#21036=VERTEX_POINT('',#107344);
#21037=VERTEX_POINT('',#107346);
#21038=VERTEX_POINT('',#107350);
#21039=VERTEX_POINT('',#107351);
#21040=VERTEX_POINT('',#107353);
#21041=VERTEX_POINT('',#107355);
#21042=VERTEX_POINT('',#107357);
#21043=VERTEX_POINT('',#107359);
#21044=VERTEX_POINT('',#107363);
#21045=VERTEX_POINT('',#107365);
#21046=VERTEX_POINT('',#107369);
#21047=VERTEX_POINT('',#107371);
#21048=VERTEX_POINT('',#107375);
#21049=VERTEX_POINT('',#107377);
#21050=VERTEX_POINT('',#107381);
#21051=VERTEX_POINT('',#107383);
#21052=VERTEX_POINT('',#107387);
#21053=VERTEX_POINT('',#107389);
#21054=VERTEX_POINT('',#107391);
#21055=VERTEX_POINT('',#107393);
#21056=VERTEX_POINT('',#107395);
#21057=VERTEX_POINT('',#107397);
#21058=VERTEX_POINT('',#107402);
#21059=VERTEX_POINT('',#107404);
#21060=VERTEX_POINT('',#107408);
#21061=VERTEX_POINT('',#107411);
#21062=VERTEX_POINT('',#107413);
#21063=VERTEX_POINT('',#107417);
#21064=VERTEX_POINT('',#107418);
#21065=VERTEX_POINT('',#107420);
#21066=VERTEX_POINT('',#107423);
#21067=VERTEX_POINT('',#107425);
#21068=VERTEX_POINT('',#107427);
#21069=VERTEX_POINT('',#107431);
#21070=VERTEX_POINT('',#107432);
#21071=VERTEX_POINT('',#107434);
#21072=VERTEX_POINT('',#107436);
#21073=VERTEX_POINT('',#107440);
#21074=VERTEX_POINT('',#107441);
#21075=VERTEX_POINT('',#107443);
#21076=VERTEX_POINT('',#107445);
#21077=VERTEX_POINT('',#107447);
#21078=VERTEX_POINT('',#107449);
#21079=VERTEX_POINT('',#107454);
#21080=VERTEX_POINT('',#107456);
#21081=VERTEX_POINT('',#107459);
#21082=VERTEX_POINT('',#107461);
#21083=VERTEX_POINT('',#107463);
#21084=VERTEX_POINT('',#107465);
#21085=VERTEX_POINT('',#107467);
#21086=VERTEX_POINT('',#107469);
#21087=VERTEX_POINT('',#107474);
#21088=VERTEX_POINT('',#107475);
#21089=VERTEX_POINT('',#107477);
#21090=VERTEX_POINT('',#107483);
#21091=VERTEX_POINT('',#107484);
#21092=VERTEX_POINT('',#107486);
#21093=VERTEX_POINT('',#107489);
#21094=VERTEX_POINT('',#107493);
#21095=VERTEX_POINT('',#107494);
#21096=VERTEX_POINT('',#107496);
#21097=VERTEX_POINT('',#107498);
#21098=VERTEX_POINT('',#107503);
#21099=VERTEX_POINT('',#107505);
#21100=VERTEX_POINT('',#107507);
#21101=VERTEX_POINT('',#107509);
#21102=VERTEX_POINT('',#107511);
#21103=VERTEX_POINT('',#107513);
#21104=VERTEX_POINT('',#107515);
#21105=VERTEX_POINT('',#107517);
#21106=VERTEX_POINT('',#107521);
#21107=VERTEX_POINT('',#107526);
#21108=VERTEX_POINT('',#107530);
#21109=VERTEX_POINT('',#107532);
#21110=VERTEX_POINT('',#107536);
#21111=VERTEX_POINT('',#107537);
#21112=VERTEX_POINT('',#107539);
#21113=VERTEX_POINT('',#107541);
#21114=VERTEX_POINT('',#107543);
#21115=VERTEX_POINT('',#107545);
#21116=VERTEX_POINT('',#107549);
#21117=VERTEX_POINT('',#107550);
#21118=VERTEX_POINT('',#107552);
#21119=VERTEX_POINT('',#107554);
#21120=VERTEX_POINT('',#107556);
#21121=VERTEX_POINT('',#107558);
#21122=VERTEX_POINT('',#107560);
#21123=VERTEX_POINT('',#107562);
#21124=VERTEX_POINT('',#107565);
#21125=VERTEX_POINT('',#107566);
#21126=VERTEX_POINT('',#107568);
#21127=VERTEX_POINT('',#107570);
#21128=VERTEX_POINT('',#107572);
#21129=VERTEX_POINT('',#107574);
#21130=VERTEX_POINT('',#107576);
#21131=VERTEX_POINT('',#107578);
#21132=VERTEX_POINT('',#107582);
#21133=VERTEX_POINT('',#107584);
#21134=VERTEX_POINT('',#107586);
#21135=VERTEX_POINT('',#107588);
#21136=VERTEX_POINT('',#107590);
#21137=VERTEX_POINT('',#107592);
#21138=VERTEX_POINT('',#107594);
#21139=VERTEX_POINT('',#107596);
#21140=VERTEX_POINT('',#107598);
#21141=VERTEX_POINT('',#107600);
#21142=VERTEX_POINT('',#107602);
#21143=VERTEX_POINT('',#107604);
#21144=VERTEX_POINT('',#107606);
#21145=VERTEX_POINT('',#107608);
#21146=VERTEX_POINT('',#107610);
#21147=VERTEX_POINT('',#107612);
#21148=VERTEX_POINT('',#107614);
#21149=VERTEX_POINT('',#107616);
#21150=VERTEX_POINT('',#107618);
#21151=VERTEX_POINT('',#107620);
#21152=VERTEX_POINT('',#107622);
#21153=VERTEX_POINT('',#107624);
#21154=VERTEX_POINT('',#107627);
#21155=VERTEX_POINT('',#107629);
#21156=VERTEX_POINT('',#107631);
#21157=VERTEX_POINT('',#107636);
#21158=VERTEX_POINT('',#107638);
#21159=VERTEX_POINT('',#107644);
#21160=VERTEX_POINT('',#107649);
#21161=VERTEX_POINT('',#107650);
#21162=VERTEX_POINT('',#107657);
#21163=VERTEX_POINT('',#107660);
#21164=VERTEX_POINT('',#107664);
#21165=VERTEX_POINT('',#107666);
#21166=VERTEX_POINT('',#107671);
#21167=VERTEX_POINT('',#107675);
#21168=VERTEX_POINT('',#107679);
#21169=VERTEX_POINT('',#107705);
#21170=VERTEX_POINT('',#107709);
#21171=VERTEX_POINT('',#107713);
#21172=VERTEX_POINT('',#107717);
#21173=VERTEX_POINT('',#107721);
#21174=VERTEX_POINT('',#107725);
#21175=VERTEX_POINT('',#107729);
#21176=VERTEX_POINT('',#107733);
#21177=VERTEX_POINT('',#107742);
#21178=VERTEX_POINT('',#107746);
#21179=VERTEX_POINT('',#107750);
#21180=VERTEX_POINT('',#107756);
#21181=VERTEX_POINT('',#107757);
#21182=VERTEX_POINT('',#107762);
#21183=VERTEX_POINT('',#107763);
#21184=VERTEX_POINT('',#107769);
#21185=VERTEX_POINT('',#107794);
#21186=VERTEX_POINT('',#107796);
#21187=VERTEX_POINT('',#107800);
#21188=VERTEX_POINT('',#107804);
#21189=VERTEX_POINT('',#107808);
#21190=VERTEX_POINT('',#107812);
#21191=VERTEX_POINT('',#107816);
#21192=VERTEX_POINT('',#107820);
#21193=VERTEX_POINT('',#107830);
#21194=VERTEX_POINT('',#107832);
#21195=VERTEX_POINT('',#107834);
#21196=VERTEX_POINT('',#107836);
#21197=VERTEX_POINT('',#107842);
#21198=VERTEX_POINT('',#107850);
#21199=VERTEX_POINT('',#107861);
#21200=VERTEX_POINT('',#107862);
#21201=VERTEX_POINT('',#107867);
#21202=VERTEX_POINT('',#107868);
#27819=EDGE_CURVE('',#21005,#21005,#17097,.T.);
#27820=EDGE_CURVE('',#21005,#21006,#11405,.T.);
#27821=EDGE_CURVE('',#21006,#21007,#17098,.T.);
#27822=EDGE_CURVE('',#21007,#21008,#11406,.T.);
#27823=EDGE_CURVE('',#21009,#21008,#17099,.T.);
#27824=EDGE_CURVE('',#21009,#21010,#11407,.T.);
#27825=EDGE_CURVE('',#21010,#21010,#17100,.T.);
#27826=EDGE_CURVE('',#21011,#21009,#17101,.T.);
#27827=EDGE_CURVE('',#21012,#21011,#11408,.T.);
#27828=EDGE_CURVE('',#21012,#21006,#17102,.T.);
#27829=EDGE_CURVE('',#21013,#21013,#17103,.T.);
#27830=EDGE_CURVE('',#21013,#21014,#11409,.T.);
#27831=EDGE_CURVE('',#21014,#21014,#17104,.T.);
#27832=EDGE_CURVE('',#21015,#21015,#2195,.F.);
#27833=EDGE_CURVE('',#21016,#21016,#17105,.T.);
#27834=EDGE_CURVE('',#21016,#21017,#11410,.T.);
#27835=EDGE_CURVE('',#21017,#21017,#17106,.T.);
#27836=EDGE_CURVE('',#21018,#21019,#17107,.T.);
#27837=EDGE_CURVE('',#21020,#21018,#11411,.T.);
#27838=EDGE_CURVE('',#21020,#21021,#17108,.T.);
#27839=EDGE_CURVE('',#21019,#21021,#11412,.T.);
#27840=EDGE_CURVE('',#21022,#21022,#17109,.T.);
#27841=EDGE_CURVE('',#21022,#21023,#11413,.T.);
#27842=EDGE_CURVE('',#21023,#21023,#17110,.T.);
#27843=EDGE_CURVE('',#21024,#21025,#17111,.T.);
#27844=EDGE_CURVE('',#21025,#21026,#11414,.T.);
#27845=EDGE_CURVE('',#21026,#21026,#17112,.T.);
#27846=EDGE_CURVE('',#21025,#21027,#17113,.T.);
#27847=EDGE_CURVE('',#21027,#21028,#2196,.F.);
#27848=EDGE_CURVE('',#21029,#21028,#17114,.T.);
#27849=EDGE_CURVE('',#21030,#21029,#17115,.T.);
#27850=EDGE_CURVE('',#21030,#21024,#2197,.F.);
#27851=EDGE_CURVE('',#21026,#21031,#11415,.T.);
#27852=EDGE_CURVE('',#21031,#21031,#17116,.T.);
#27853=EDGE_CURVE('',#21032,#21032,#17117,.T.);
#27854=EDGE_CURVE('',#21032,#21033,#11416,.T.);
#27855=EDGE_CURVE('',#21033,#21033,#17118,.T.);
#27856=EDGE_CURVE('',#21034,#21035,#17119,.T.);
#27857=EDGE_CURVE('',#21036,#21034,#11417,.T.);
#27858=EDGE_CURVE('',#21037,#21036,#17120,.T.);
#27859=EDGE_CURVE('',#21037,#21035,#11418,.T.);
#27860=EDGE_CURVE('',#21038,#21039,#17121,.T.);
#27861=EDGE_CURVE('',#21038,#21040,#11419,.T.);
#27862=EDGE_CURVE('',#21040,#21041,#17122,.T.);
#27863=EDGE_CURVE('',#21042,#21041,#11420,.T.);
#27864=EDGE_CURVE('',#21043,#21042,#17123,.T.);
#27865=EDGE_CURVE('',#21039,#21043,#11421,.T.);
#27866=EDGE_CURVE('',#21044,#21044,#17124,.T.);
#27867=EDGE_CURVE('',#21044,#21045,#11422,.T.);
#27868=EDGE_CURVE('',#21045,#21045,#17125,.T.);
#27869=EDGE_CURVE('',#21046,#21046,#17126,.T.);
#27870=EDGE_CURVE('',#21046,#21047,#11423,.T.);
#27871=EDGE_CURVE('',#21047,#21047,#17127,.T.);
#27872=EDGE_CURVE('',#21048,#21048,#17128,.T.);
#27873=EDGE_CURVE('',#21048,#21049,#11424,.T.);
#27874=EDGE_CURVE('',#21049,#21049,#17129,.T.);
#27875=EDGE_CURVE('',#21050,#21050,#17130,.T.);
#27876=EDGE_CURVE('',#21050,#21051,#11425,.T.);
#27877=EDGE_CURVE('',#21051,#21051,#17131,.T.);
#27878=EDGE_CURVE('',#21052,#21052,#17132,.T.);
#27879=EDGE_CURVE('',#21052,#21053,#11426,.T.);
#27880=EDGE_CURVE('',#21053,#21054,#17133,.T.);
#27881=EDGE_CURVE('',#21055,#21054,#11427,.T.);
#27882=EDGE_CURVE('',#21056,#21055,#17134,.T.);
#27883=EDGE_CURVE('',#21056,#21057,#11428,.T.);
#27884=EDGE_CURVE('',#21057,#21057,#17135,.T.);
#27885=EDGE_CURVE('',#21056,#21053,#11429,.T.);
#27886=EDGE_CURVE('',#21058,#21058,#17136,.T.);
#27887=EDGE_CURVE('',#21058,#21059,#11430,.T.);
#27888=EDGE_CURVE('',#21059,#21059,#17137,.T.);
#27889=EDGE_CURVE('',#21029,#21060,#11431,.T.);
#27890=EDGE_CURVE('',#21060,#21060,#17138,.T.);
#27891=EDGE_CURVE('',#21028,#21061,#11432,.T.);
#27892=EDGE_CURVE('',#21061,#21062,#17139,.T.);
#27893=EDGE_CURVE('',#21062,#21030,#11433,.T.);
#27894=EDGE_CURVE('',#21063,#21064,#17140,.T.);
#27895=EDGE_CURVE('',#21063,#21065,#11434,.T.);
#27896=EDGE_CURVE('',#21065,#21020,#17141,.T.);
#27897=EDGE_CURVE('',#21066,#21018,#17142,.T.);
#27898=EDGE_CURVE('',#21066,#21067,#11435,.T.);
#27899=EDGE_CURVE('',#21068,#21067,#17143,.T.);
#27900=EDGE_CURVE('',#21064,#21068,#11436,.T.);
#27901=EDGE_CURVE('',#21069,#21070,#11437,.T.);
#27902=EDGE_CURVE('',#21069,#21071,#11438,.T.);
#27903=EDGE_CURVE('',#21071,#21072,#11439,.T.);
#27904=EDGE_CURVE('',#21072,#21070,#11440,.T.);
#27905=EDGE_CURVE('',#21073,#21074,#11441,.T.);
#27906=EDGE_CURVE('',#21073,#21075,#17144,.T.);
#27907=EDGE_CURVE('',#21076,#21075,#11442,.T.);
#27908=EDGE_CURVE('',#21076,#21077,#17145,.T.);
#27909=EDGE_CURVE('',#21078,#21077,#11443,.T.);
#27910=EDGE_CURVE('',#21024,#21078,#17146,.T.);
#27911=EDGE_CURVE('',#21062,#21074,#17147,.T.);
#27912=EDGE_CURVE('',#21074,#21079,#11444,.T.);
#27913=EDGE_CURVE('',#21080,#21061,#17148,.T.);
#27914=EDGE_CURVE('',#21054,#21080,#11445,.T.);
#27915=EDGE_CURVE('',#21081,#21053,#11446,.T.);
#27916=EDGE_CURVE('',#21082,#21081,#17149,.T.);
#27917=EDGE_CURVE('',#21082,#21083,#11447,.T.);
#27918=EDGE_CURVE('',#21083,#21084,#11448,.T.);
#27919=EDGE_CURVE('',#21084,#21085,#11449,.T.);
#27920=EDGE_CURVE('',#21085,#21086,#11450,.T.);
#27921=EDGE_CURVE('',#21086,#21077,#11451,.T.);
#27922=EDGE_CURVE('',#21079,#21076,#11452,.T.);
#27923=EDGE_CURVE('',#21087,#21088,#11453,.T.);
#27924=EDGE_CURVE('',#21088,#21089,#11454,.T.);
#27925=EDGE_CURVE('',#21069,#21089,#11455,.T.);
#27926=EDGE_CURVE('',#21075,#21069,#11456,.T.);
#27927=EDGE_CURVE('',#21087,#21073,#11457,.T.);
#27928=EDGE_CURVE('',#21090,#21091,#11458,.T.);
#27929=EDGE_CURVE('',#21090,#21092,#11459,.T.);
#27930=EDGE_CURVE('',#21092,#21070,#11460,.T.);
#27931=EDGE_CURVE('',#21070,#21093,#11461,.T.);
#27932=EDGE_CURVE('',#21093,#21091,#11462,.T.);
#27933=EDGE_CURVE('',#21094,#21095,#11463,.T.);
#27934=EDGE_CURVE('',#21095,#21096,#11464,.T.);
#27935=EDGE_CURVE('',#21097,#21096,#11465,.T.);
#27936=EDGE_CURVE('',#21097,#21094,#11466,.T.);
#27937=EDGE_CURVE('',#21043,#21065,#17150,.T.);
#27938=EDGE_CURVE('',#21042,#21098,#11467,.T.);
#27939=EDGE_CURVE('',#21098,#21099,#17151,.T.);
#27940=EDGE_CURVE('',#21099,#21100,#11468,.T.);
#27941=EDGE_CURVE('',#21100,#21101,#17152,.T.);
#27942=EDGE_CURVE('',#21101,#21102,#11469,.T.);
#27943=EDGE_CURVE('',#21102,#21103,#17153,.T.);
#27944=EDGE_CURVE('',#21103,#21104,#11470,.T.);
#27945=EDGE_CURVE('',#21105,#21104,#17154,.T.);
#27946=EDGE_CURVE('',#21021,#21105,#17155,.T.);
#27947=EDGE_CURVE('',#21106,#21105,#11471,.T.);
#27948=EDGE_CURVE('',#21036,#21106,#17156,.T.);
#27949=EDGE_CURVE('',#21019,#21034,#17157,.T.);
#27950=EDGE_CURVE('',#21107,#21027,#17158,.T.);
#27951=EDGE_CURVE('',#21107,#21080,#11472,.T.);
#27952=EDGE_CURVE('',#21108,#21037,#11473,.T.);
#27953=EDGE_CURVE('',#21108,#21109,#11474,.T.);
#27954=EDGE_CURVE('',#21109,#21035,#11475,.T.);
#27955=EDGE_CURVE('',#21110,#21111,#11476,.T.);
#27956=EDGE_CURVE('',#21112,#21111,#11477,.T.);
#27957=EDGE_CURVE('',#21113,#21112,#11478,.T.);
#27958=EDGE_CURVE('',#21113,#21114,#11479,.T.);
#27959=EDGE_CURVE('',#21115,#21114,#11480,.T.);
#27960=EDGE_CURVE('',#21110,#21115,#11481,.T.);
#27961=EDGE_CURVE('',#21116,#21117,#11482,.T.);
#27962=EDGE_CURVE('',#21117,#21118,#11483,.T.);
#27963=EDGE_CURVE('',#21118,#21119,#11484,.T.);
#27964=EDGE_CURVE('',#21119,#21120,#11485,.T.);
#27965=EDGE_CURVE('',#21120,#21121,#11486,.T.);
#27966=EDGE_CURVE('',#21121,#21122,#11487,.T.);
#27967=EDGE_CURVE('',#21122,#21123,#11488,.T.);
#27968=EDGE_CURVE('',#21123,#21116,#11489,.T.);
#27969=EDGE_CURVE('',#21124,#21125,#11490,.T.);
#27970=EDGE_CURVE('',#21126,#21124,#11491,.T.);
#27971=EDGE_CURVE('',#21127,#21126,#11492,.T.);
#27972=EDGE_CURVE('',#21128,#21127,#11493,.T.);
#27973=EDGE_CURVE('',#21129,#21128,#11494,.T.);
#27974=EDGE_CURVE('',#21130,#21129,#11495,.T.);
#27975=EDGE_CURVE('',#21131,#21130,#11496,.T.);
#27976=EDGE_CURVE('',#21125,#21131,#11497,.T.);
#27977=EDGE_CURVE('',#21132,#21109,#11498,.T.);
#27978=EDGE_CURVE('',#21132,#21133,#11499,.T.);
#27979=EDGE_CURVE('',#21134,#21133,#11500,.T.);
#27980=EDGE_CURVE('',#21135,#21134,#11501,.T.);
#27981=EDGE_CURVE('',#21136,#21135,#11502,.T.);
#27982=EDGE_CURVE('',#21137,#21136,#11503,.T.);
#27983=EDGE_CURVE('',#21138,#21137,#11504,.T.);
#27984=EDGE_CURVE('',#21139,#21138,#11505,.T.);
#27985=EDGE_CURVE('',#21140,#21139,#11506,.T.);
#27986=EDGE_CURVE('',#21141,#21140,#17159,.T.);
#27987=EDGE_CURVE('',#21142,#21141,#11507,.T.);
#27988=EDGE_CURVE('',#21143,#21142,#17160,.T.);
#27989=EDGE_CURVE('',#21144,#21143,#11508,.T.);
#27990=EDGE_CURVE('',#21145,#21144,#17161,.T.);
#27991=EDGE_CURVE('',#21146,#21145,#11509,.T.);
#27992=EDGE_CURVE('',#21146,#21147,#11510,.T.);
#27993=EDGE_CURVE('',#21148,#21147,#11511,.T.);
#27994=EDGE_CURVE('',#21149,#21148,#17162,.T.);
#27995=EDGE_CURVE('',#21150,#21149,#11512,.T.);
#27996=EDGE_CURVE('',#21151,#21150,#17163,.T.);
#27997=EDGE_CURVE('',#21152,#21151,#11513,.T.);
#27998=EDGE_CURVE('',#21153,#21152,#17164,.T.);
#27999=EDGE_CURVE('',#21041,#21153,#11514,.T.);
#28000=EDGE_CURVE('',#21154,#21040,#11515,.T.);
#28001=EDGE_CURVE('',#21155,#21154,#17165,.T.);
#28002=EDGE_CURVE('',#21156,#21155,#11516,.T.);
#28003=EDGE_CURVE('',#21111,#21156,#17166,.T.);
#28004=EDGE_CURVE('',#21110,#21066,#17167,.T.);
#28005=EDGE_CURVE('',#21157,#21134,#11517,.T.);
#28006=EDGE_CURVE('',#21157,#21158,#11518,.T.);
#28007=EDGE_CURVE('',#21158,#21135,#11519,.T.);
#28008=EDGE_CURVE('',#21095,#21093,#11520,.T.);
#28009=EDGE_CURVE('',#21094,#21157,#11521,.T.);
#28010=EDGE_CURVE('',#21159,#21133,#11522,.T.);
#28011=EDGE_CURVE('',#21089,#21159,#11523,.T.);
#28012=EDGE_CURVE('',#21091,#21088,#11524,.T.);
#28013=EDGE_CURVE('',#21160,#21161,#11525,.T.);
#28014=EDGE_CURVE('',#21160,#21159,#11526,.T.);
#28015=EDGE_CURVE('',#21133,#21161,#11527,.T.);
#28016=EDGE_CURVE('',#21072,#21096,#11528,.T.);
#28017=EDGE_CURVE('',#21071,#21160,#11529,.T.);
#28018=EDGE_CURVE('',#21162,#21161,#11530,.T.);
#28019=EDGE_CURVE('',#21086,#21162,#11531,.T.);
#28020=EDGE_CURVE('',#21163,#21085,#11532,.T.);
#28021=EDGE_CURVE('',#21163,#21097,#11533,.T.);
#28022=EDGE_CURVE('',#21164,#21084,#11534,.T.);
#28023=EDGE_CURVE('',#21164,#21165,#11535,.T.);
#28024=EDGE_CURVE('',#21165,#21163,#11536,.T.);
#28025=EDGE_CURVE('',#21083,#21139,#11537,.T.);
#28026=EDGE_CURVE('',#21166,#21138,#11538,.T.);
#28027=EDGE_CURVE('',#21166,#21164,#11539,.T.);
#28028=EDGE_CURVE('',#21167,#21137,#11540,.T.);
#28029=EDGE_CURVE('',#21167,#21166,#11541,.T.);
#28030=EDGE_CURVE('',#21168,#21136,#11542,.T.);
#28031=EDGE_CURVE('',#21168,#21167,#11543,.T.);
#28032=EDGE_CURVE('',#21158,#21168,#11544,.T.);
#28033=EDGE_CURVE('',#21158,#21121,#11545,.T.);
#28034=EDGE_CURVE('',#21122,#21157,#11546,.T.);
#28035=EDGE_CURVE('',#21123,#21094,#11547,.T.);
#28036=EDGE_CURVE('',#21168,#21120,#11548,.T.);
#28037=EDGE_CURVE('',#21116,#21097,#11549,.T.);
#28038=EDGE_CURVE('',#21167,#21119,#11550,.T.);
#28039=EDGE_CURVE('',#21117,#21165,#11551,.T.);
#28040=EDGE_CURVE('',#21166,#21118,#11552,.T.);
#28041=EDGE_CURVE('',#21162,#21146,#11553,.T.);
#28042=EDGE_CURVE('',#21169,#21145,#11554,.T.);
#28043=EDGE_CURVE('',#21169,#21078,#11555,.T.);
#28044=EDGE_CURVE('',#21170,#21144,#11556,.T.);
#28045=EDGE_CURVE('',#21170,#21169,#17168,.T.);
#28046=EDGE_CURVE('',#21171,#21143,#11557,.T.);
#28047=EDGE_CURVE('',#21171,#21170,#11558,.T.);
#28048=EDGE_CURVE('',#21172,#21142,#11559,.T.);
#28049=EDGE_CURVE('',#21172,#21171,#17169,.T.);
#28050=EDGE_CURVE('',#21173,#21141,#11560,.T.);
#28051=EDGE_CURVE('',#21173,#21172,#11561,.T.);
#28052=EDGE_CURVE('',#21174,#21140,#11562,.T.);
#28053=EDGE_CURVE('',#21174,#21173,#17170,.T.);
#28054=EDGE_CURVE('',#21082,#21175,#11563,.T.);
#28055=EDGE_CURVE('',#21175,#21174,#11564,.T.);
#28056=EDGE_CURVE('',#21176,#21081,#11565,.T.);
#28057=EDGE_CURVE('',#21175,#21176,#17171,.T.);
#28058=EDGE_CURVE('',#21176,#21056,#11566,.T.);
#28059=EDGE_CURVE('',#21055,#21107,#11567,.T.);
#28060=EDGE_CURVE('',#21177,#21038,#11568,.T.);
#28061=EDGE_CURVE('',#21177,#21154,#11569,.T.);
#28062=EDGE_CURVE('',#21178,#21177,#17172,.T.);
#28063=EDGE_CURVE('',#21178,#21155,#11570,.T.);
#28064=EDGE_CURVE('',#21179,#21178,#11571,.T.);
#28065=EDGE_CURVE('',#21179,#21156,#11572,.T.);
#28066=EDGE_CURVE('',#21112,#21179,#17173,.T.);
#28067=EDGE_CURVE('',#21180,#21181,#11573,.T.);
#28068=EDGE_CURVE('',#21181,#21132,#11574,.T.);
#28069=EDGE_CURVE('',#21180,#21108,#11575,.T.);
#28070=EDGE_CURVE('',#21182,#21183,#11576,.T.);
#28071=EDGE_CURVE('',#21183,#21181,#11577,.T.);
#28072=EDGE_CURVE('',#21182,#21180,#11578,.T.);
#28073=EDGE_CURVE('',#21147,#21183,#11579,.T.);
#28074=EDGE_CURVE('',#21184,#21182,#11580,.T.);
#28075=EDGE_CURVE('',#21184,#21104,#11581,.T.);
#28076=EDGE_CURVE('',#21103,#21148,#11582,.T.);
#28077=EDGE_CURVE('',#21102,#21149,#11583,.T.);
#28078=EDGE_CURVE('',#21101,#21150,#11584,.T.);
#28079=EDGE_CURVE('',#21100,#21151,#11585,.T.);
#28080=EDGE_CURVE('',#21099,#21152,#11586,.T.);
#28081=EDGE_CURVE('',#21098,#21153,#11587,.T.);
#28082=EDGE_CURVE('',#21067,#21115,#17174,.T.);
#28083=EDGE_CURVE('',#21114,#21068,#11588,.T.);
#28084=EDGE_CURVE('',#21185,#21124,#11589,.T.);
#28085=EDGE_CURVE('',#21186,#21185,#11590,.T.);
#28086=EDGE_CURVE('',#21186,#21126,#11591,.T.);
#28087=EDGE_CURVE('',#21187,#21186,#11592,.T.);
#28088=EDGE_CURVE('',#21187,#21127,#11593,.T.);
#28089=EDGE_CURVE('',#21188,#21187,#11594,.T.);
#28090=EDGE_CURVE('',#21188,#21128,#11595,.T.);
#28091=EDGE_CURVE('',#21189,#21188,#11596,.T.);
#28092=EDGE_CURVE('',#21189,#21129,#11597,.T.);
#28093=EDGE_CURVE('',#21190,#21189,#11598,.T.);
#28094=EDGE_CURVE('',#21190,#21130,#11599,.T.);
#28095=EDGE_CURVE('',#21191,#21190,#11600,.T.);
#28096=EDGE_CURVE('',#21191,#21131,#11601,.T.);
#28097=EDGE_CURVE('',#21192,#21191,#11602,.T.);
#28098=EDGE_CURVE('',#21192,#21125,#11603,.T.);
#28099=EDGE_CURVE('',#21185,#21192,#11604,.T.);
#28100=EDGE_CURVE('',#21106,#21184,#17175,.T.);
#28101=EDGE_CURVE('',#21193,#21113,#11605,.T.);
#28102=EDGE_CURVE('',#21193,#21194,#11606,.T.);
#28103=EDGE_CURVE('',#21194,#21195,#11607,.T.);
#28104=EDGE_CURVE('',#21195,#21196,#11608,.T.);
#28105=EDGE_CURVE('',#21064,#21196,#11609,.T.);
#28106=EDGE_CURVE('',#21039,#21063,#17176,.T.);
#28107=EDGE_CURVE('',#21193,#21197,#11610,.T.);
#28108=EDGE_CURVE('',#21197,#21196,#11611,.T.);
#28109=EDGE_CURVE('',#21087,#21090,#11612,.T.);
#28110=EDGE_CURVE('',#21194,#21198,#11613,.T.);
#28111=EDGE_CURVE('',#21198,#21195,#11614,.T.);
#28112=EDGE_CURVE('',#21198,#21197,#11615,.T.);
#28113=EDGE_CURVE('',#21079,#21092,#11616,.T.);
#28114=EDGE_CURVE('',#21199,#21200,#17177,.T.);
#28115=EDGE_CURVE('',#21011,#21199,#11617,.T.);
#28116=EDGE_CURVE('',#21200,#21008,#11618,.T.);
#28117=EDGE_CURVE('',#21201,#21202,#17178,.T.);
#28118=EDGE_CURVE('',#21199,#21201,#11619,.T.);
#28119=EDGE_CURVE('',#21202,#21200,#11620,.T.);
#28120=EDGE_CURVE('',#21201,#21012,#11621,.T.);
#28121=EDGE_CURVE('',#21007,#21202,#11622,.T.);
#41354=ORIENTED_EDGE('',*,*,#27819,.F.);
#41355=ORIENTED_EDGE('',*,*,#27820,.T.);
#41356=ORIENTED_EDGE('',*,*,#27821,.T.);
#41357=ORIENTED_EDGE('',*,*,#27822,.T.);
#41358=ORIENTED_EDGE('',*,*,#27823,.F.);
#41359=ORIENTED_EDGE('',*,*,#27824,.T.);
#41360=ORIENTED_EDGE('',*,*,#27825,.T.);
#41361=ORIENTED_EDGE('',*,*,#27824,.F.);
#41362=ORIENTED_EDGE('',*,*,#27826,.F.);
#41363=ORIENTED_EDGE('',*,*,#27827,.F.);
#41364=ORIENTED_EDGE('',*,*,#27828,.T.);
#41365=ORIENTED_EDGE('',*,*,#27820,.F.);
#41366=ORIENTED_EDGE('',*,*,#27829,.T.);
#41367=ORIENTED_EDGE('',*,*,#27830,.T.);
#41368=ORIENTED_EDGE('',*,*,#27831,.F.);
#41369=ORIENTED_EDGE('',*,*,#27830,.F.);
#41370=ORIENTED_EDGE('',*,*,#27832,.F.);
#41371=ORIENTED_EDGE('',*,*,#27833,.T.);
#41372=ORIENTED_EDGE('',*,*,#27834,.T.);
#41373=ORIENTED_EDGE('',*,*,#27835,.T.);
#41374=ORIENTED_EDGE('',*,*,#27834,.F.);
#41375=ORIENTED_EDGE('',*,*,#27836,.F.);
#41376=ORIENTED_EDGE('',*,*,#27837,.F.);
#41377=ORIENTED_EDGE('',*,*,#27838,.T.);
#41378=ORIENTED_EDGE('',*,*,#27839,.F.);
#41379=ORIENTED_EDGE('',*,*,#27840,.F.);
#41380=ORIENTED_EDGE('',*,*,#27841,.T.);
#41381=ORIENTED_EDGE('',*,*,#27842,.T.);
#41382=ORIENTED_EDGE('',*,*,#27841,.F.);
#41383=ORIENTED_EDGE('',*,*,#27832,.T.);
#41384=ORIENTED_EDGE('',*,*,#27843,.T.);
#41385=ORIENTED_EDGE('',*,*,#27844,.T.);
#41386=ORIENTED_EDGE('',*,*,#27845,.T.);
#41387=ORIENTED_EDGE('',*,*,#27844,.F.);
#41388=ORIENTED_EDGE('',*,*,#27846,.T.);
#41389=ORIENTED_EDGE('',*,*,#27847,.T.);
#41390=ORIENTED_EDGE('',*,*,#27848,.F.);
#41391=ORIENTED_EDGE('',*,*,#27849,.F.);
#41392=ORIENTED_EDGE('',*,*,#27850,.T.);
#41393=ORIENTED_EDGE('',*,*,#27845,.F.);
#41394=ORIENTED_EDGE('',*,*,#27851,.T.);
#41395=ORIENTED_EDGE('',*,*,#27852,.T.);
#41396=ORIENTED_EDGE('',*,*,#27851,.F.);
#41397=ORIENTED_EDGE('',*,*,#27853,.T.);
#41398=ORIENTED_EDGE('',*,*,#27854,.T.);
#41399=ORIENTED_EDGE('',*,*,#27855,.T.);
#41400=ORIENTED_EDGE('',*,*,#27854,.F.);
#41401=ORIENTED_EDGE('',*,*,#27856,.F.);
#41402=ORIENTED_EDGE('',*,*,#27857,.F.);
#41403=ORIENTED_EDGE('',*,*,#27858,.F.);
#41404=ORIENTED_EDGE('',*,*,#27859,.T.);
#41405=ORIENTED_EDGE('',*,*,#27860,.F.);
#41406=ORIENTED_EDGE('',*,*,#27861,.T.);
#41407=ORIENTED_EDGE('',*,*,#27862,.T.);
#41408=ORIENTED_EDGE('',*,*,#27863,.F.);
#41409=ORIENTED_EDGE('',*,*,#27864,.F.);
#41410=ORIENTED_EDGE('',*,*,#27865,.F.);
#41411=ORIENTED_EDGE('',*,*,#27866,.F.);
#41412=ORIENTED_EDGE('',*,*,#27867,.T.);
#41413=ORIENTED_EDGE('',*,*,#27868,.T.);
#41414=ORIENTED_EDGE('',*,*,#27867,.F.);
#41415=ORIENTED_EDGE('',*,*,#27869,.F.);
#41416=ORIENTED_EDGE('',*,*,#27870,.T.);
#41417=ORIENTED_EDGE('',*,*,#27871,.T.);
#41418=ORIENTED_EDGE('',*,*,#27870,.F.);
#41419=ORIENTED_EDGE('',*,*,#27872,.F.);
#41420=ORIENTED_EDGE('',*,*,#27873,.T.);
#41421=ORIENTED_EDGE('',*,*,#27874,.T.);
#41422=ORIENTED_EDGE('',*,*,#27873,.F.);
#41423=ORIENTED_EDGE('',*,*,#27875,.T.);
#41424=ORIENTED_EDGE('',*,*,#27876,.T.);
#41425=ORIENTED_EDGE('',*,*,#27877,.F.);
#41426=ORIENTED_EDGE('',*,*,#27876,.F.);
#41427=ORIENTED_EDGE('',*,*,#27878,.T.);
#41428=ORIENTED_EDGE('',*,*,#27879,.T.);
#41429=ORIENTED_EDGE('',*,*,#27880,.T.);
#41430=ORIENTED_EDGE('',*,*,#27881,.F.);
#41431=ORIENTED_EDGE('',*,*,#27882,.F.);
#41432=ORIENTED_EDGE('',*,*,#27883,.T.);
#41433=ORIENTED_EDGE('',*,*,#27884,.F.);
#41434=ORIENTED_EDGE('',*,*,#27883,.F.);
#41435=ORIENTED_EDGE('',*,*,#27885,.T.);
#41436=ORIENTED_EDGE('',*,*,#27879,.F.);
#41437=ORIENTED_EDGE('',*,*,#27886,.T.);
#41438=ORIENTED_EDGE('',*,*,#27887,.T.);
#41439=ORIENTED_EDGE('',*,*,#27888,.F.);
#41440=ORIENTED_EDGE('',*,*,#27887,.F.);
#41441=ORIENTED_EDGE('',*,*,#27849,.T.);
#41442=ORIENTED_EDGE('',*,*,#27889,.T.);
#41443=ORIENTED_EDGE('',*,*,#27890,.F.);
#41444=ORIENTED_EDGE('',*,*,#27889,.F.);
#41445=ORIENTED_EDGE('',*,*,#27848,.T.);
#41446=ORIENTED_EDGE('',*,*,#27891,.T.);
#41447=ORIENTED_EDGE('',*,*,#27892,.T.);
#41448=ORIENTED_EDGE('',*,*,#27893,.T.);
#41449=ORIENTED_EDGE('',*,*,#27894,.F.);
#41450=ORIENTED_EDGE('',*,*,#27895,.T.);
#41451=ORIENTED_EDGE('',*,*,#27896,.T.);
#41452=ORIENTED_EDGE('',*,*,#27837,.T.);
#41453=ORIENTED_EDGE('',*,*,#27897,.F.);
#41454=ORIENTED_EDGE('',*,*,#27898,.T.);
#41455=ORIENTED_EDGE('',*,*,#27899,.F.);
#41456=ORIENTED_EDGE('',*,*,#27900,.F.);
#41457=ORIENTED_EDGE('',*,*,#27901,.F.);
#41458=ORIENTED_EDGE('',*,*,#27902,.T.);
#41459=ORIENTED_EDGE('',*,*,#27903,.T.);
#41460=ORIENTED_EDGE('',*,*,#27904,.T.);
#41461=ORIENTED_EDGE('',*,*,#27905,.F.);
#41462=ORIENTED_EDGE('',*,*,#27906,.T.);
#41463=ORIENTED_EDGE('',*,*,#27907,.F.);
#41464=ORIENTED_EDGE('',*,*,#27908,.T.);
#41465=ORIENTED_EDGE('',*,*,#27909,.F.);
#41466=ORIENTED_EDGE('',*,*,#27910,.F.);
#41467=ORIENTED_EDGE('',*,*,#27850,.F.);
#41468=ORIENTED_EDGE('',*,*,#27893,.F.);
#41469=ORIENTED_EDGE('',*,*,#27911,.T.);
#41470=ORIENTED_EDGE('',*,*,#27912,.F.);
#41471=ORIENTED_EDGE('',*,*,#27911,.F.);
#41472=ORIENTED_EDGE('',*,*,#27892,.F.);
#41473=ORIENTED_EDGE('',*,*,#27913,.F.);
#41474=ORIENTED_EDGE('',*,*,#27914,.F.);
#41475=ORIENTED_EDGE('',*,*,#27880,.F.);
#41476=ORIENTED_EDGE('',*,*,#27915,.F.);
#41477=ORIENTED_EDGE('',*,*,#27916,.F.);
#41478=ORIENTED_EDGE('',*,*,#27917,.T.);
#41479=ORIENTED_EDGE('',*,*,#27918,.T.);
#41480=ORIENTED_EDGE('',*,*,#27919,.T.);
#41481=ORIENTED_EDGE('',*,*,#27920,.T.);
#41482=ORIENTED_EDGE('',*,*,#27921,.T.);
#41483=ORIENTED_EDGE('',*,*,#27908,.F.);
#41484=ORIENTED_EDGE('',*,*,#27922,.F.);
#41485=ORIENTED_EDGE('',*,*,#27923,.T.);
#41486=ORIENTED_EDGE('',*,*,#27924,.T.);
#41487=ORIENTED_EDGE('',*,*,#27925,.F.);
#41488=ORIENTED_EDGE('',*,*,#27926,.F.);
#41489=ORIENTED_EDGE('',*,*,#27906,.F.);
#41490=ORIENTED_EDGE('',*,*,#27927,.F.);
#41491=ORIENTED_EDGE('',*,*,#27928,.F.);
#41492=ORIENTED_EDGE('',*,*,#27929,.T.);
#41493=ORIENTED_EDGE('',*,*,#27930,.T.);
#41494=ORIENTED_EDGE('',*,*,#27931,.T.);
#41495=ORIENTED_EDGE('',*,*,#27932,.T.);
#41496=ORIENTED_EDGE('',*,*,#27933,.T.);
#41497=ORIENTED_EDGE('',*,*,#27934,.T.);
#41498=ORIENTED_EDGE('',*,*,#27935,.F.);
#41499=ORIENTED_EDGE('',*,*,#27936,.T.);
#41500=ORIENTED_EDGE('',*,*,#27937,.F.);
#41501=ORIENTED_EDGE('',*,*,#27864,.T.);
#41502=ORIENTED_EDGE('',*,*,#27938,.T.);
#41503=ORIENTED_EDGE('',*,*,#27939,.T.);
#41504=ORIENTED_EDGE('',*,*,#27940,.T.);
#41505=ORIENTED_EDGE('',*,*,#27941,.T.);
#41506=ORIENTED_EDGE('',*,*,#27942,.T.);
#41507=ORIENTED_EDGE('',*,*,#27943,.T.);
#41508=ORIENTED_EDGE('',*,*,#27944,.T.);
#41509=ORIENTED_EDGE('',*,*,#27945,.F.);
#41510=ORIENTED_EDGE('',*,*,#27946,.F.);
#41511=ORIENTED_EDGE('',*,*,#27838,.F.);
#41512=ORIENTED_EDGE('',*,*,#27896,.F.);
#41513=ORIENTED_EDGE('',*,*,#27946,.T.);
#41514=ORIENTED_EDGE('',*,*,#27947,.F.);
#41515=ORIENTED_EDGE('',*,*,#27948,.F.);
#41516=ORIENTED_EDGE('',*,*,#27857,.T.);
#41517=ORIENTED_EDGE('',*,*,#27949,.F.);
#41518=ORIENTED_EDGE('',*,*,#27839,.T.);
#41519=ORIENTED_EDGE('',*,*,#27847,.F.);
#41520=ORIENTED_EDGE('',*,*,#27950,.F.);
#41521=ORIENTED_EDGE('',*,*,#27951,.T.);
#41522=ORIENTED_EDGE('',*,*,#27913,.T.);
#41523=ORIENTED_EDGE('',*,*,#27891,.F.);
#41524=ORIENTED_EDGE('',*,*,#27859,.F.);
#41525=ORIENTED_EDGE('',*,*,#27952,.F.);
#41526=ORIENTED_EDGE('',*,*,#27953,.T.);
#41527=ORIENTED_EDGE('',*,*,#27954,.T.);
#41528=ORIENTED_EDGE('',*,*,#27955,.T.);
#41529=ORIENTED_EDGE('',*,*,#27956,.F.);
#41530=ORIENTED_EDGE('',*,*,#27957,.F.);
#41531=ORIENTED_EDGE('',*,*,#27958,.T.);
#41532=ORIENTED_EDGE('',*,*,#27959,.F.);
#41533=ORIENTED_EDGE('',*,*,#27960,.F.);
#41534=ORIENTED_EDGE('',*,*,#27961,.T.);
#41535=ORIENTED_EDGE('',*,*,#27962,.T.);
#41536=ORIENTED_EDGE('',*,*,#27963,.T.);
#41537=ORIENTED_EDGE('',*,*,#27964,.T.);
#41538=ORIENTED_EDGE('',*,*,#27965,.T.);
#41539=ORIENTED_EDGE('',*,*,#27966,.T.);
#41540=ORIENTED_EDGE('',*,*,#27967,.T.);
#41541=ORIENTED_EDGE('',*,*,#27968,.T.);
#41542=ORIENTED_EDGE('',*,*,#27969,.F.);
#41543=ORIENTED_EDGE('',*,*,#27970,.F.);
#41544=ORIENTED_EDGE('',*,*,#27971,.F.);
#41545=ORIENTED_EDGE('',*,*,#27972,.F.);
#41546=ORIENTED_EDGE('',*,*,#27973,.F.);
#41547=ORIENTED_EDGE('',*,*,#27974,.F.);
#41548=ORIENTED_EDGE('',*,*,#27975,.F.);
#41549=ORIENTED_EDGE('',*,*,#27976,.F.);
#41550=ORIENTED_EDGE('',*,*,#27874,.F.);
#41551=ORIENTED_EDGE('',*,*,#27871,.F.);
#41552=ORIENTED_EDGE('',*,*,#27868,.F.);
#41553=ORIENTED_EDGE('',*,*,#27897,.T.);
#41554=ORIENTED_EDGE('',*,*,#27836,.T.);
#41555=ORIENTED_EDGE('',*,*,#27949,.T.);
#41556=ORIENTED_EDGE('',*,*,#27856,.T.);
#41557=ORIENTED_EDGE('',*,*,#27954,.F.);
#41558=ORIENTED_EDGE('',*,*,#27977,.F.);
#41559=ORIENTED_EDGE('',*,*,#27978,.T.);
#41560=ORIENTED_EDGE('',*,*,#27979,.F.);
#41561=ORIENTED_EDGE('',*,*,#27980,.F.);
#41562=ORIENTED_EDGE('',*,*,#27981,.F.);
#41563=ORIENTED_EDGE('',*,*,#27982,.F.);
#41564=ORIENTED_EDGE('',*,*,#27983,.F.);
#41565=ORIENTED_EDGE('',*,*,#27984,.F.);
#41566=ORIENTED_EDGE('',*,*,#27985,.F.);
#41567=ORIENTED_EDGE('',*,*,#27986,.F.);
#41568=ORIENTED_EDGE('',*,*,#27987,.F.);
#41569=ORIENTED_EDGE('',*,*,#27988,.F.);
#41570=ORIENTED_EDGE('',*,*,#27989,.F.);
#41571=ORIENTED_EDGE('',*,*,#27990,.F.);
#41572=ORIENTED_EDGE('',*,*,#27991,.F.);
#41573=ORIENTED_EDGE('',*,*,#27992,.T.);
#41574=ORIENTED_EDGE('',*,*,#27993,.F.);
#41575=ORIENTED_EDGE('',*,*,#27994,.F.);
#41576=ORIENTED_EDGE('',*,*,#27995,.F.);
#41577=ORIENTED_EDGE('',*,*,#27996,.F.);
#41578=ORIENTED_EDGE('',*,*,#27997,.F.);
#41579=ORIENTED_EDGE('',*,*,#27998,.F.);
#41580=ORIENTED_EDGE('',*,*,#27999,.F.);
#41581=ORIENTED_EDGE('',*,*,#27862,.F.);
#41582=ORIENTED_EDGE('',*,*,#28000,.F.);
#41583=ORIENTED_EDGE('',*,*,#28001,.F.);
#41584=ORIENTED_EDGE('',*,*,#28002,.F.);
#41585=ORIENTED_EDGE('',*,*,#28003,.F.);
#41586=ORIENTED_EDGE('',*,*,#27955,.F.);
#41587=ORIENTED_EDGE('',*,*,#28004,.T.);
#41588=ORIENTED_EDGE('',*,*,#27852,.F.);
#41589=ORIENTED_EDGE('',*,*,#27884,.T.);
#41590=ORIENTED_EDGE('',*,*,#27888,.T.);
#41591=ORIENTED_EDGE('',*,*,#27877,.T.);
#41592=ORIENTED_EDGE('',*,*,#27853,.F.);
#41593=ORIENTED_EDGE('',*,*,#27833,.F.);
#41594=ORIENTED_EDGE('',*,*,#28005,.F.);
#41595=ORIENTED_EDGE('',*,*,#28006,.T.);
#41596=ORIENTED_EDGE('',*,*,#28007,.T.);
#41597=ORIENTED_EDGE('',*,*,#27980,.T.);
#41598=ORIENTED_EDGE('',*,*,#27932,.F.);
#41599=ORIENTED_EDGE('',*,*,#28008,.F.);
#41600=ORIENTED_EDGE('',*,*,#27933,.F.);
#41601=ORIENTED_EDGE('',*,*,#28009,.T.);
#41602=ORIENTED_EDGE('',*,*,#28005,.T.);
#41603=ORIENTED_EDGE('',*,*,#27979,.T.);
#41604=ORIENTED_EDGE('',*,*,#28010,.F.);
#41605=ORIENTED_EDGE('',*,*,#28011,.F.);
#41606=ORIENTED_EDGE('',*,*,#27924,.F.);
#41607=ORIENTED_EDGE('',*,*,#28012,.F.);
#41608=ORIENTED_EDGE('',*,*,#28013,.F.);
#41609=ORIENTED_EDGE('',*,*,#28014,.T.);
#41610=ORIENTED_EDGE('',*,*,#28010,.T.);
#41611=ORIENTED_EDGE('',*,*,#28015,.T.);
#41612=ORIENTED_EDGE('',*,*,#27935,.T.);
#41613=ORIENTED_EDGE('',*,*,#28016,.F.);
#41614=ORIENTED_EDGE('',*,*,#27903,.F.);
#41615=ORIENTED_EDGE('',*,*,#28017,.T.);
#41616=ORIENTED_EDGE('',*,*,#28013,.T.);
#41617=ORIENTED_EDGE('',*,*,#28018,.F.);
#41618=ORIENTED_EDGE('',*,*,#28019,.F.);
#41619=ORIENTED_EDGE('',*,*,#27920,.F.);
#41620=ORIENTED_EDGE('',*,*,#28020,.F.);
#41621=ORIENTED_EDGE('',*,*,#28021,.T.);
#41622=ORIENTED_EDGE('',*,*,#27831,.T.);
#41623=ORIENTED_EDGE('',*,*,#28020,.T.);
#41624=ORIENTED_EDGE('',*,*,#27919,.F.);
#41625=ORIENTED_EDGE('',*,*,#28022,.F.);
#41626=ORIENTED_EDGE('',*,*,#28023,.T.);
#41627=ORIENTED_EDGE('',*,*,#28024,.T.);
#41628=ORIENTED_EDGE('',*,*,#28022,.T.);
#41629=ORIENTED_EDGE('',*,*,#27918,.F.);
#41630=ORIENTED_EDGE('',*,*,#28025,.T.);
#41631=ORIENTED_EDGE('',*,*,#27984,.T.);
#41632=ORIENTED_EDGE('',*,*,#28026,.F.);
#41633=ORIENTED_EDGE('',*,*,#28027,.T.);
#41634=ORIENTED_EDGE('',*,*,#28028,.F.);
#41635=ORIENTED_EDGE('',*,*,#28029,.T.);
#41636=ORIENTED_EDGE('',*,*,#28026,.T.);
#41637=ORIENTED_EDGE('',*,*,#27983,.T.);
#41638=ORIENTED_EDGE('',*,*,#28030,.F.);
#41639=ORIENTED_EDGE('',*,*,#28031,.T.);
#41640=ORIENTED_EDGE('',*,*,#28028,.T.);
#41641=ORIENTED_EDGE('',*,*,#27982,.T.);
#41642=ORIENTED_EDGE('',*,*,#28007,.F.);
#41643=ORIENTED_EDGE('',*,*,#28032,.T.);
#41644=ORIENTED_EDGE('',*,*,#28030,.T.);
#41645=ORIENTED_EDGE('',*,*,#27981,.T.);
#41646=ORIENTED_EDGE('',*,*,#27825,.F.);
#41647=ORIENTED_EDGE('',*,*,#28033,.F.);
#41648=ORIENTED_EDGE('',*,*,#28006,.F.);
#41649=ORIENTED_EDGE('',*,*,#28034,.F.);
#41650=ORIENTED_EDGE('',*,*,#27966,.F.);
#41651=ORIENTED_EDGE('',*,*,#28034,.T.);
#41652=ORIENTED_EDGE('',*,*,#28009,.F.);
#41653=ORIENTED_EDGE('',*,*,#28035,.F.);
#41654=ORIENTED_EDGE('',*,*,#27967,.F.);
#41655=ORIENTED_EDGE('',*,*,#28033,.T.);
#41656=ORIENTED_EDGE('',*,*,#27965,.F.);
#41657=ORIENTED_EDGE('',*,*,#28036,.F.);
#41658=ORIENTED_EDGE('',*,*,#28032,.F.);
#41659=ORIENTED_EDGE('',*,*,#28035,.T.);
#41660=ORIENTED_EDGE('',*,*,#27936,.F.);
#41661=ORIENTED_EDGE('',*,*,#28037,.F.);
#41662=ORIENTED_EDGE('',*,*,#27968,.F.);
#41663=ORIENTED_EDGE('',*,*,#28036,.T.);
#41664=ORIENTED_EDGE('',*,*,#27964,.F.);
#41665=ORIENTED_EDGE('',*,*,#28038,.F.);
#41666=ORIENTED_EDGE('',*,*,#28031,.F.);
#41667=ORIENTED_EDGE('',*,*,#28021,.F.);
#41668=ORIENTED_EDGE('',*,*,#28024,.F.);
#41669=ORIENTED_EDGE('',*,*,#28039,.F.);
#41670=ORIENTED_EDGE('',*,*,#27961,.F.);
#41671=ORIENTED_EDGE('',*,*,#28037,.T.);
#41672=ORIENTED_EDGE('',*,*,#28038,.T.);
#41673=ORIENTED_EDGE('',*,*,#27963,.F.);
#41674=ORIENTED_EDGE('',*,*,#28040,.F.);
#41675=ORIENTED_EDGE('',*,*,#28029,.F.);
#41676=ORIENTED_EDGE('',*,*,#28023,.F.);
#41677=ORIENTED_EDGE('',*,*,#28027,.F.);
#41678=ORIENTED_EDGE('',*,*,#28040,.T.);
#41679=ORIENTED_EDGE('',*,*,#27962,.F.);
#41680=ORIENTED_EDGE('',*,*,#28039,.T.);
#41681=ORIENTED_EDGE('',*,*,#27872,.T.);
#41682=ORIENTED_EDGE('',*,*,#27875,.F.);
#41683=ORIENTED_EDGE('',*,*,#27869,.T.);
#41684=ORIENTED_EDGE('',*,*,#27878,.F.);
#41685=ORIENTED_EDGE('',*,*,#27866,.T.);
#41686=ORIENTED_EDGE('',*,*,#27886,.F.);
#41687=ORIENTED_EDGE('',*,*,#28019,.T.);
#41688=ORIENTED_EDGE('',*,*,#28041,.T.);
#41689=ORIENTED_EDGE('',*,*,#27991,.T.);
#41690=ORIENTED_EDGE('',*,*,#28042,.F.);
#41691=ORIENTED_EDGE('',*,*,#28043,.T.);
#41692=ORIENTED_EDGE('',*,*,#27909,.T.);
#41693=ORIENTED_EDGE('',*,*,#27921,.F.);
#41694=ORIENTED_EDGE('',*,*,#28044,.F.);
#41695=ORIENTED_EDGE('',*,*,#28045,.T.);
#41696=ORIENTED_EDGE('',*,*,#28042,.T.);
#41697=ORIENTED_EDGE('',*,*,#27990,.T.);
#41698=ORIENTED_EDGE('',*,*,#28046,.F.);
#41699=ORIENTED_EDGE('',*,*,#28047,.T.);
#41700=ORIENTED_EDGE('',*,*,#28044,.T.);
#41701=ORIENTED_EDGE('',*,*,#27989,.T.);
#41702=ORIENTED_EDGE('',*,*,#28048,.F.);
#41703=ORIENTED_EDGE('',*,*,#28049,.T.);
#41704=ORIENTED_EDGE('',*,*,#28046,.T.);
#41705=ORIENTED_EDGE('',*,*,#27988,.T.);
#41706=ORIENTED_EDGE('',*,*,#28050,.F.);
#41707=ORIENTED_EDGE('',*,*,#28051,.T.);
#41708=ORIENTED_EDGE('',*,*,#28048,.T.);
#41709=ORIENTED_EDGE('',*,*,#27987,.T.);
#41710=ORIENTED_EDGE('',*,*,#28052,.F.);
#41711=ORIENTED_EDGE('',*,*,#28053,.T.);
#41712=ORIENTED_EDGE('',*,*,#28050,.T.);
#41713=ORIENTED_EDGE('',*,*,#27986,.T.);
#41714=ORIENTED_EDGE('',*,*,#27917,.F.);
#41715=ORIENTED_EDGE('',*,*,#28054,.T.);
#41716=ORIENTED_EDGE('',*,*,#28055,.T.);
#41717=ORIENTED_EDGE('',*,*,#28052,.T.);
#41718=ORIENTED_EDGE('',*,*,#27985,.T.);
#41719=ORIENTED_EDGE('',*,*,#28025,.F.);
#41720=ORIENTED_EDGE('',*,*,#27916,.T.);
#41721=ORIENTED_EDGE('',*,*,#28056,.F.);
#41722=ORIENTED_EDGE('',*,*,#28057,.F.);
#41723=ORIENTED_EDGE('',*,*,#28054,.F.);
#41724=ORIENTED_EDGE('',*,*,#27843,.F.);
#41725=ORIENTED_EDGE('',*,*,#27910,.T.);
#41726=ORIENTED_EDGE('',*,*,#28043,.F.);
#41727=ORIENTED_EDGE('',*,*,#28045,.F.);
#41728=ORIENTED_EDGE('',*,*,#28047,.F.);
#41729=ORIENTED_EDGE('',*,*,#28049,.F.);
#41730=ORIENTED_EDGE('',*,*,#28051,.F.);
#41731=ORIENTED_EDGE('',*,*,#28053,.F.);
#41732=ORIENTED_EDGE('',*,*,#28055,.F.);
#41733=ORIENTED_EDGE('',*,*,#28057,.T.);
#41734=ORIENTED_EDGE('',*,*,#28058,.T.);
#41735=ORIENTED_EDGE('',*,*,#27882,.T.);
#41736=ORIENTED_EDGE('',*,*,#28059,.T.);
#41737=ORIENTED_EDGE('',*,*,#27950,.T.);
#41738=ORIENTED_EDGE('',*,*,#27846,.F.);
#41739=ORIENTED_EDGE('',*,*,#27915,.T.);
#41740=ORIENTED_EDGE('',*,*,#27885,.F.);
#41741=ORIENTED_EDGE('',*,*,#28058,.F.);
#41742=ORIENTED_EDGE('',*,*,#28056,.T.);
#41743=ORIENTED_EDGE('',*,*,#27914,.T.);
#41744=ORIENTED_EDGE('',*,*,#27951,.F.);
#41745=ORIENTED_EDGE('',*,*,#28059,.F.);
#41746=ORIENTED_EDGE('',*,*,#27881,.T.);
#41747=ORIENTED_EDGE('',*,*,#28000,.T.);
#41748=ORIENTED_EDGE('',*,*,#27861,.F.);
#41749=ORIENTED_EDGE('',*,*,#28060,.F.);
#41750=ORIENTED_EDGE('',*,*,#28061,.T.);
#41751=ORIENTED_EDGE('',*,*,#28001,.T.);
#41752=ORIENTED_EDGE('',*,*,#28061,.F.);
#41753=ORIENTED_EDGE('',*,*,#28062,.F.);
#41754=ORIENTED_EDGE('',*,*,#28063,.T.);
#41755=ORIENTED_EDGE('',*,*,#28002,.T.);
#41756=ORIENTED_EDGE('',*,*,#28063,.F.);
#41757=ORIENTED_EDGE('',*,*,#28064,.F.);
#41758=ORIENTED_EDGE('',*,*,#28065,.T.);
#41759=ORIENTED_EDGE('',*,*,#28003,.T.);
#41760=ORIENTED_EDGE('',*,*,#28065,.F.);
#41761=ORIENTED_EDGE('',*,*,#28066,.F.);
#41762=ORIENTED_EDGE('',*,*,#27956,.T.);
#41763=ORIENTED_EDGE('',*,*,#28067,.T.);
#41764=ORIENTED_EDGE('',*,*,#28068,.T.);
#41765=ORIENTED_EDGE('',*,*,#27977,.T.);
#41766=ORIENTED_EDGE('',*,*,#27953,.F.);
#41767=ORIENTED_EDGE('',*,*,#28069,.F.);
#41768=ORIENTED_EDGE('',*,*,#28070,.T.);
#41769=ORIENTED_EDGE('',*,*,#28071,.T.);
#41770=ORIENTED_EDGE('',*,*,#28067,.F.);
#41771=ORIENTED_EDGE('',*,*,#28072,.F.);
#41772=ORIENTED_EDGE('',*,*,#27993,.T.);
#41773=ORIENTED_EDGE('',*,*,#28073,.T.);
#41774=ORIENTED_EDGE('',*,*,#28070,.F.);
#41775=ORIENTED_EDGE('',*,*,#28074,.F.);
#41776=ORIENTED_EDGE('',*,*,#28075,.T.);
#41777=ORIENTED_EDGE('',*,*,#27944,.F.);
#41778=ORIENTED_EDGE('',*,*,#28076,.T.);
#41779=ORIENTED_EDGE('',*,*,#27994,.T.);
#41780=ORIENTED_EDGE('',*,*,#28076,.F.);
#41781=ORIENTED_EDGE('',*,*,#27943,.F.);
#41782=ORIENTED_EDGE('',*,*,#28077,.T.);
#41783=ORIENTED_EDGE('',*,*,#27995,.T.);
#41784=ORIENTED_EDGE('',*,*,#28077,.F.);
#41785=ORIENTED_EDGE('',*,*,#27942,.F.);
#41786=ORIENTED_EDGE('',*,*,#28078,.T.);
#41787=ORIENTED_EDGE('',*,*,#27996,.T.);
#41788=ORIENTED_EDGE('',*,*,#28078,.F.);
#41789=ORIENTED_EDGE('',*,*,#27941,.F.);
#41790=ORIENTED_EDGE('',*,*,#28079,.T.);
#41791=ORIENTED_EDGE('',*,*,#27997,.T.);
#41792=ORIENTED_EDGE('',*,*,#28079,.F.);
#41793=ORIENTED_EDGE('',*,*,#27940,.F.);
#41794=ORIENTED_EDGE('',*,*,#28080,.T.);
#41795=ORIENTED_EDGE('',*,*,#27998,.T.);
#41796=ORIENTED_EDGE('',*,*,#28080,.F.);
#41797=ORIENTED_EDGE('',*,*,#27939,.F.);
#41798=ORIENTED_EDGE('',*,*,#28081,.T.);
#41799=ORIENTED_EDGE('',*,*,#27999,.T.);
#41800=ORIENTED_EDGE('',*,*,#28081,.F.);
#41801=ORIENTED_EDGE('',*,*,#27938,.F.);
#41802=ORIENTED_EDGE('',*,*,#27863,.T.);
#41803=ORIENTED_EDGE('',*,*,#27978,.F.);
#41804=ORIENTED_EDGE('',*,*,#28068,.F.);
#41805=ORIENTED_EDGE('',*,*,#28071,.F.);
#41806=ORIENTED_EDGE('',*,*,#28073,.F.);
#41807=ORIENTED_EDGE('',*,*,#27992,.F.);
#41808=ORIENTED_EDGE('',*,*,#28041,.F.);
#41809=ORIENTED_EDGE('',*,*,#28018,.T.);
#41810=ORIENTED_EDGE('',*,*,#28015,.F.);
#41811=ORIENTED_EDGE('',*,*,#28004,.F.);
#41812=ORIENTED_EDGE('',*,*,#27960,.T.);
#41813=ORIENTED_EDGE('',*,*,#28082,.F.);
#41814=ORIENTED_EDGE('',*,*,#27898,.F.);
#41815=ORIENTED_EDGE('',*,*,#27855,.F.);
#41816=ORIENTED_EDGE('',*,*,#27899,.T.);
#41817=ORIENTED_EDGE('',*,*,#28082,.T.);
#41818=ORIENTED_EDGE('',*,*,#27959,.T.);
#41819=ORIENTED_EDGE('',*,*,#28083,.T.);
#41820=ORIENTED_EDGE('',*,*,#27890,.T.);
#41821=ORIENTED_EDGE('',*,*,#27842,.F.);
#41822=ORIENTED_EDGE('',*,*,#27840,.T.);
#41823=ORIENTED_EDGE('',*,*,#27835,.F.);
#41824=ORIENTED_EDGE('',*,*,#27970,.T.);
#41825=ORIENTED_EDGE('',*,*,#28084,.F.);
#41826=ORIENTED_EDGE('',*,*,#28085,.F.);
#41827=ORIENTED_EDGE('',*,*,#28086,.T.);
#41828=ORIENTED_EDGE('',*,*,#27971,.T.);
#41829=ORIENTED_EDGE('',*,*,#28086,.F.);
#41830=ORIENTED_EDGE('',*,*,#28087,.F.);
#41831=ORIENTED_EDGE('',*,*,#28088,.T.);
#41832=ORIENTED_EDGE('',*,*,#27972,.T.);
#41833=ORIENTED_EDGE('',*,*,#28088,.F.);
#41834=ORIENTED_EDGE('',*,*,#28089,.F.);
#41835=ORIENTED_EDGE('',*,*,#28090,.T.);
#41836=ORIENTED_EDGE('',*,*,#27973,.T.);
#41837=ORIENTED_EDGE('',*,*,#28090,.F.);
#41838=ORIENTED_EDGE('',*,*,#28091,.F.);
#41839=ORIENTED_EDGE('',*,*,#28092,.T.);
#41840=ORIENTED_EDGE('',*,*,#27974,.T.);
#41841=ORIENTED_EDGE('',*,*,#28092,.F.);
#41842=ORIENTED_EDGE('',*,*,#28093,.F.);
#41843=ORIENTED_EDGE('',*,*,#28094,.T.);
#41844=ORIENTED_EDGE('',*,*,#27975,.T.);
#41845=ORIENTED_EDGE('',*,*,#28094,.F.);
#41846=ORIENTED_EDGE('',*,*,#28095,.F.);
#41847=ORIENTED_EDGE('',*,*,#28096,.T.);
#41848=ORIENTED_EDGE('',*,*,#27976,.T.);
#41849=ORIENTED_EDGE('',*,*,#28096,.F.);
#41850=ORIENTED_EDGE('',*,*,#28097,.F.);
#41851=ORIENTED_EDGE('',*,*,#28098,.T.);
#41852=ORIENTED_EDGE('',*,*,#27969,.T.);
#41853=ORIENTED_EDGE('',*,*,#28098,.F.);
#41854=ORIENTED_EDGE('',*,*,#28099,.F.);
#41855=ORIENTED_EDGE('',*,*,#28084,.T.);
#41856=ORIENTED_EDGE('',*,*,#28085,.T.);
#41857=ORIENTED_EDGE('',*,*,#28099,.T.);
#41858=ORIENTED_EDGE('',*,*,#28097,.T.);
#41859=ORIENTED_EDGE('',*,*,#28095,.T.);
#41860=ORIENTED_EDGE('',*,*,#28093,.T.);
#41861=ORIENTED_EDGE('',*,*,#28091,.T.);
#41862=ORIENTED_EDGE('',*,*,#28089,.T.);
#41863=ORIENTED_EDGE('',*,*,#28087,.T.);
#41864=ORIENTED_EDGE('',*,*,#27945,.T.);
#41865=ORIENTED_EDGE('',*,*,#28075,.F.);
#41866=ORIENTED_EDGE('',*,*,#28100,.F.);
#41867=ORIENTED_EDGE('',*,*,#27947,.T.);
#41868=ORIENTED_EDGE('',*,*,#28100,.T.);
#41869=ORIENTED_EDGE('',*,*,#28074,.T.);
#41870=ORIENTED_EDGE('',*,*,#28072,.T.);
#41871=ORIENTED_EDGE('',*,*,#28069,.T.);
#41872=ORIENTED_EDGE('',*,*,#27952,.T.);
#41873=ORIENTED_EDGE('',*,*,#27858,.T.);
#41874=ORIENTED_EDGE('',*,*,#27948,.T.);
#41875=ORIENTED_EDGE('',*,*,#28101,.F.);
#41876=ORIENTED_EDGE('',*,*,#28102,.T.);
#41877=ORIENTED_EDGE('',*,*,#28103,.T.);
#41878=ORIENTED_EDGE('',*,*,#28104,.T.);
#41879=ORIENTED_EDGE('',*,*,#28105,.F.);
#41880=ORIENTED_EDGE('',*,*,#27900,.T.);
#41881=ORIENTED_EDGE('',*,*,#28083,.F.);
#41882=ORIENTED_EDGE('',*,*,#27958,.F.);
#41883=ORIENTED_EDGE('',*,*,#27937,.T.);
#41884=ORIENTED_EDGE('',*,*,#27895,.F.);
#41885=ORIENTED_EDGE('',*,*,#28106,.F.);
#41886=ORIENTED_EDGE('',*,*,#27865,.T.);
#41887=ORIENTED_EDGE('',*,*,#28107,.F.);
#41888=ORIENTED_EDGE('',*,*,#28101,.T.);
#41889=ORIENTED_EDGE('',*,*,#27957,.T.);
#41890=ORIENTED_EDGE('',*,*,#28066,.T.);
#41891=ORIENTED_EDGE('',*,*,#28064,.T.);
#41892=ORIENTED_EDGE('',*,*,#28062,.T.);
#41893=ORIENTED_EDGE('',*,*,#28060,.T.);
#41894=ORIENTED_EDGE('',*,*,#27860,.T.);
#41895=ORIENTED_EDGE('',*,*,#28106,.T.);
#41896=ORIENTED_EDGE('',*,*,#27894,.T.);
#41897=ORIENTED_EDGE('',*,*,#28105,.T.);
#41898=ORIENTED_EDGE('',*,*,#28108,.F.);
#41899=ORIENTED_EDGE('',*,*,#28008,.T.);
#41900=ORIENTED_EDGE('',*,*,#27931,.F.);
#41901=ORIENTED_EDGE('',*,*,#27904,.F.);
#41902=ORIENTED_EDGE('',*,*,#28016,.T.);
#41903=ORIENTED_EDGE('',*,*,#27934,.F.);
#41904=ORIENTED_EDGE('',*,*,#28017,.F.);
#41905=ORIENTED_EDGE('',*,*,#27902,.F.);
#41906=ORIENTED_EDGE('',*,*,#27925,.T.);
#41907=ORIENTED_EDGE('',*,*,#28011,.T.);
#41908=ORIENTED_EDGE('',*,*,#28014,.F.);
#41909=ORIENTED_EDGE('',*,*,#27923,.F.);
#41910=ORIENTED_EDGE('',*,*,#28109,.T.);
#41911=ORIENTED_EDGE('',*,*,#27928,.T.);
#41912=ORIENTED_EDGE('',*,*,#28012,.T.);
#41913=ORIENTED_EDGE('',*,*,#28103,.F.);
#41914=ORIENTED_EDGE('',*,*,#28110,.T.);
#41915=ORIENTED_EDGE('',*,*,#28111,.T.);
#41916=ORIENTED_EDGE('',*,*,#28110,.F.);
#41917=ORIENTED_EDGE('',*,*,#28102,.F.);
#41918=ORIENTED_EDGE('',*,*,#28107,.T.);
#41919=ORIENTED_EDGE('',*,*,#28112,.F.);
#41920=ORIENTED_EDGE('',*,*,#28108,.T.);
#41921=ORIENTED_EDGE('',*,*,#28104,.F.);
#41922=ORIENTED_EDGE('',*,*,#28111,.F.);
#41923=ORIENTED_EDGE('',*,*,#28112,.T.);
#41924=ORIENTED_EDGE('',*,*,#27905,.T.);
#41925=ORIENTED_EDGE('',*,*,#27912,.T.);
#41926=ORIENTED_EDGE('',*,*,#28113,.T.);
#41927=ORIENTED_EDGE('',*,*,#27929,.F.);
#41928=ORIENTED_EDGE('',*,*,#28109,.F.);
#41929=ORIENTED_EDGE('',*,*,#27927,.T.);
#41930=ORIENTED_EDGE('',*,*,#27907,.T.);
#41931=ORIENTED_EDGE('',*,*,#27926,.T.);
#41932=ORIENTED_EDGE('',*,*,#27901,.T.);
#41933=ORIENTED_EDGE('',*,*,#27930,.F.);
#41934=ORIENTED_EDGE('',*,*,#28113,.F.);
#41935=ORIENTED_EDGE('',*,*,#27922,.T.);
#41936=ORIENTED_EDGE('',*,*,#27819,.T.);
#41937=ORIENTED_EDGE('',*,*,#27829,.F.);
#41938=ORIENTED_EDGE('',*,*,#28114,.F.);
#41939=ORIENTED_EDGE('',*,*,#28115,.F.);
#41940=ORIENTED_EDGE('',*,*,#27826,.T.);
#41941=ORIENTED_EDGE('',*,*,#27823,.T.);
#41942=ORIENTED_EDGE('',*,*,#28116,.F.);
#41943=ORIENTED_EDGE('',*,*,#28117,.F.);
#41944=ORIENTED_EDGE('',*,*,#28118,.F.);
#41945=ORIENTED_EDGE('',*,*,#28114,.T.);
#41946=ORIENTED_EDGE('',*,*,#28119,.F.);
#41947=ORIENTED_EDGE('',*,*,#27828,.F.);
#41948=ORIENTED_EDGE('',*,*,#28120,.F.);
#41949=ORIENTED_EDGE('',*,*,#28117,.T.);
#41950=ORIENTED_EDGE('',*,*,#28121,.F.);
#41951=ORIENTED_EDGE('',*,*,#27821,.F.);
#41952=ORIENTED_EDGE('',*,*,#28118,.T.);
#41953=ORIENTED_EDGE('',*,*,#28120,.T.);
#41954=ORIENTED_EDGE('',*,*,#27827,.T.);
#41955=ORIENTED_EDGE('',*,*,#28115,.T.);
#41956=ORIENTED_EDGE('',*,*,#28119,.T.);
#41957=ORIENTED_EDGE('',*,*,#28116,.T.);
#41958=ORIENTED_EDGE('',*,*,#27822,.F.);
#41959=ORIENTED_EDGE('',*,*,#28121,.T.);
#42580=CYLINDRICAL_SURFACE('',#50174,0.008);
#42581=CYLINDRICAL_SURFACE('',#50181,0.002125);
#42582=CYLINDRICAL_SURFACE('',#50184,0.003);
#42583=CYLINDRICAL_SURFACE('',#50187,0.005);
#42584=CYLINDRICAL_SURFACE('',#50190,0.0025);
#42585=CYLINDRICAL_SURFACE('',#50199,0.01125);
#42586=CYLINDRICAL_SURFACE('',#50201,0.0015);
#42587=CYLINDRICAL_SURFACE('',#50204,0.0036);
#42588=CYLINDRICAL_SURFACE('',#50207,0.0037);
#42589=CYLINDRICAL_SURFACE('',#50211,0.002825);
#42590=CYLINDRICAL_SURFACE('',#50214,0.002825);
#42591=CYLINDRICAL_SURFACE('',#50217,0.002825);
#42592=CYLINDRICAL_SURFACE('',#50220,0.0016);
#42593=CYLINDRICAL_SURFACE('',#50223,0.0016);
#42594=CYLINDRICAL_SURFACE('',#50228,0.0016);
#42595=CYLINDRICAL_SURFACE('',#50231,0.0059);
#42596=CYLINDRICAL_SURFACE('',#50234,0.0135);
#42597=CYLINDRICAL_SURFACE('',#50240,0.014);
#42598=CYLINDRICAL_SURFACE('',#50258,0.0135);
#42599=CYLINDRICAL_SURFACE('',#50261,0.014);
#42600=CYLINDRICAL_SURFACE('',#50297,0.003);
#42601=CYLINDRICAL_SURFACE('',#50300,0.00725);
#42602=CYLINDRICAL_SURFACE('',#50303,0.004);
#42603=CYLINDRICAL_SURFACE('',#50306,0.014);
#42604=CYLINDRICAL_SURFACE('',#50312,0.0037);
#42605=CYLINDRICAL_SURFACE('',#50315,0.0037);
#42606=CYLINDRICAL_SURFACE('',#50320,0.005);
#42607=CYLINDRICAL_SURFACE('',#50322,0.00525);
#42608=CYLINDRICAL_SURFACE('',#50324,0.00650498845854181);
#42609=CYLINDRICAL_SURFACE('',#50327,0.0036);
#42610=CYLINDRICAL_SURFACE('',#50343,0.01565);
#42611=CYLINDRICAL_SURFACE('',#50347,0.01565);
#42612=CYLINDRICAL_SURFACE('',#50361,0.006);
#45427=ADVANCED_FACE('',(#6572),#42580,.F.);
#45428=ADVANCED_FACE('',(#6573,#3523),#42581,.F.);
#45429=ADVANCED_FACE('',(#6574),#42582,.F.);
#45430=ADVANCED_FACE('',(#6575),#42583,.T.);
#45431=ADVANCED_FACE('',(#6576,#3524),#42584,.F.);
#45432=ADVANCED_FACE('',(#6577),#883,.F.);
#45433=ADVANCED_FACE('',(#6578),#42585,.F.);
#45434=ADVANCED_FACE('',(#6579),#42586,.F.);
#45435=ADVANCED_FACE('',(#6580),#42587,.T.);
#45436=ADVANCED_FACE('',(#6581),#42588,.T.);
#45437=ADVANCED_FACE('',(#6582),#42589,.F.);
#45438=ADVANCED_FACE('',(#6583),#42590,.F.);
#45439=ADVANCED_FACE('',(#6584),#42591,.F.);
#45440=ADVANCED_FACE('',(#6585),#42592,.F.);
#45441=ADVANCED_FACE('',(#6586),#42593,.F.);
#45442=ADVANCED_FACE('',(#6587),#42594,.F.);
#45443=ADVANCED_FACE('',(#6588),#42595,.F.);
#45444=ADVANCED_FACE('',(#6589),#42596,.T.);
#45445=ADVANCED_FACE('',(#6590),#3682,.F.);
#45446=ADVANCED_FACE('',(#6591),#42597,.F.);
#45447=ADVANCED_FACE('',(#6592),#3683,.F.);
#45448=ADVANCED_FACE('',(#6593),#3684,.F.);
#45449=ADVANCED_FACE('',(#6594),#3685,.F.);
#45450=ADVANCED_FACE('',(#6595),#3686,.F.);
#45451=ADVANCED_FACE('',(#6596),#3687,.T.);
#45452=ADVANCED_FACE('',(#6597),#42598,.T.);
#45453=ADVANCED_FACE('',(#6598),#42599,.F.);
#45454=ADVANCED_FACE('',(#6599),#3688,.F.);
#45455=ADVANCED_FACE('',(#6600),#3689,.F.);
#45456=ADVANCED_FACE('',(#6601,#3525,#3526,#3527,#3528),#3690,.F.);
#45457=ADVANCED_FACE('',(#6602,#3529,#3530,#3531,#3532,#3533,#3534),#3691,
 .T.);
#45458=ADVANCED_FACE('',(#6603),#3692,.F.);
#45459=ADVANCED_FACE('',(#6604),#3693,.F.);
#45460=ADVANCED_FACE('',(#6605),#3694,.F.);
#45461=ADVANCED_FACE('',(#6606,#3535),#3695,.F.);
#45462=ADVANCED_FACE('',(#6607),#3696,.F.);
#45463=ADVANCED_FACE('',(#6608),#3697,.F.);
#45464=ADVANCED_FACE('',(#6609),#3698,.F.);
#45465=ADVANCED_FACE('',(#6610),#3699,.F.);
#45466=ADVANCED_FACE('',(#6611,#3536),#3700,.F.);
#45467=ADVANCED_FACE('',(#6612),#3701,.F.);
#45468=ADVANCED_FACE('',(#6613),#3702,.F.);
#45469=ADVANCED_FACE('',(#6614),#3703,.F.);
#45470=ADVANCED_FACE('',(#6615),#3704,.F.);
#45471=ADVANCED_FACE('',(#6616),#3705,.F.);
#45472=ADVANCED_FACE('',(#6617),#3706,.F.);
#45473=ADVANCED_FACE('',(#6618),#3707,.F.);
#45474=ADVANCED_FACE('',(#6619),#3708,.F.);
#45475=ADVANCED_FACE('',(#6620,#3537),#3709,.T.);
#45476=ADVANCED_FACE('',(#6621,#3538),#3710,.T.);
#45477=ADVANCED_FACE('',(#6622,#3539),#3711,.T.);
#45478=ADVANCED_FACE('',(#6623),#3712,.F.);
#45479=ADVANCED_FACE('',(#6624),#42600,.F.);
#45480=ADVANCED_FACE('',(#6625),#3713,.F.);
#45481=ADVANCED_FACE('',(#6626),#42601,.T.);
#45482=ADVANCED_FACE('',(#6627),#3714,.F.);
#45483=ADVANCED_FACE('',(#6628),#42602,.F.);
#45484=ADVANCED_FACE('',(#6629),#3715,.F.);
#45485=ADVANCED_FACE('',(#6630),#42603,.F.);
#45486=ADVANCED_FACE('',(#6631),#3716,.F.);
#45487=ADVANCED_FACE('',(#6632),#3717,.F.);
#45488=ADVANCED_FACE('',(#6633),#3718,.F.);
#45489=ADVANCED_FACE('',(#6634),#3719,.F.);
#45490=ADVANCED_FACE('',(#6635),#42604,.T.);
#45491=ADVANCED_FACE('',(#6636),#3720,.F.);
#45492=ADVANCED_FACE('',(#6637),#42605,.T.);
#45493=ADVANCED_FACE('',(#6638),#3721,.F.);
#45494=ADVANCED_FACE('',(#6639),#3722,.F.);
#45495=ADVANCED_FACE('',(#6640),#3723,.F.);
#45496=ADVANCED_FACE('',(#6641),#42606,.T.);
#45497=ADVANCED_FACE('',(#6642),#3724,.F.);
#45498=ADVANCED_FACE('',(#6643),#42607,.F.);
#45499=ADVANCED_FACE('',(#6644),#3725,.F.);
#45500=ADVANCED_FACE('',(#6645),#42608,.T.);
#45501=ADVANCED_FACE('',(#6646),#3726,.F.);
#45502=ADVANCED_FACE('',(#6647),#3727,.F.);
#45503=ADVANCED_FACE('',(#6648),#42609,.T.);
#45504=ADVANCED_FACE('',(#6649),#3728,.T.);
#45505=ADVANCED_FACE('',(#6650),#3729,.F.);
#45506=ADVANCED_FACE('',(#6651,#3540),#3730,.T.);
#45507=ADVANCED_FACE('',(#6652),#3731,.T.);
#45508=ADVANCED_FACE('',(#6653),#3732,.T.);
#45509=ADVANCED_FACE('',(#6654),#3733,.F.);
#45510=ADVANCED_FACE('',(#6655),#3734,.F.);
#45511=ADVANCED_FACE('',(#6656),#3735,.F.);
#45512=ADVANCED_FACE('',(#6657),#3736,.F.);
#45513=ADVANCED_FACE('',(#6658),#3737,.F.);
#45514=ADVANCED_FACE('',(#6659),#3738,.F.);
#45515=ADVANCED_FACE('',(#6660),#3739,.F.);
#45516=ADVANCED_FACE('',(#6661),#3740,.F.);
#45517=ADVANCED_FACE('',(#6662),#3741,.F.);
#45518=ADVANCED_FACE('',(#6663),#42610,.T.);
#45519=ADVANCED_FACE('',(#6664),#3742,.T.);
#45520=ADVANCED_FACE('',(#6665),#3743,.F.);
#45521=ADVANCED_FACE('',(#6666),#42611,.T.);
#45522=ADVANCED_FACE('',(#6667),#3744,.T.);
#45523=ADVANCED_FACE('',(#6668),#3745,.F.);
#45524=ADVANCED_FACE('',(#6669),#3746,.F.);
#45525=ADVANCED_FACE('',(#6670),#3747,.F.);
#45526=ADVANCED_FACE('',(#6671),#3748,.T.);
#45527=ADVANCED_FACE('',(#6672),#3749,.F.);
#45528=ADVANCED_FACE('',(#6673),#3750,.F.);
#45529=ADVANCED_FACE('',(#6674),#3751,.T.);
#45530=ADVANCED_FACE('',(#6675),#3752,.T.);
#45531=ADVANCED_FACE('',(#6676,#3541),#3753,.F.);
#45532=ADVANCED_FACE('',(#6677),#3754,.F.);
#45533=ADVANCED_FACE('',(#6678),#42612,.F.);
#45534=ADVANCED_FACE('',(#6679),#3755,.F.);
#45535=ADVANCED_FACE('',(#6680),#3756,.F.);
#45536=ADVANCED_FACE('',(#6681),#3757,.F.);
#45546=CLOSED_SHELL('',(#45427,#45428,#45429,#45430,#45431,#45432,#45433,
#45434,#45435,#45436,#45437,#45438,#45439,#45440,#45441,#45442,#45443,#45444,
#45445,#45446,#45447,#45448,#45449,#45450,#45451,#45452,#45453,#45454,#45455,
#45456,#45457,#45458,#45459,#45460,#45461,#45462,#45463,#45464,#45465,#45466,
#45467,#45468,#45469,#45470,#45471,#45472,#45473,#45474,#45475,#45476,#45477,
#45478,#45479,#45480,#45481,#45482,#45483,#45484,#45485,#45486,#45487,#45488,
#45489,#45490,#45491,#45492,#45493,#45494,#45495,#45496,#45497,#45498,#45499,
#45500,#45501,#45502,#45503,#45504,#45505,#45506,#45507,#45508,#45509,#45510,
#45511,#45512,#45513,#45514,#45515,#45516,#45517,#45518,#45519,#45520,#45521,
#45522,#45523,#45524,#45525,#45526,#45527,#45528,#45529,#45530,#45531,#45532,
#45533,#45534,#45535,#45536));
#50173=AXIS2_PLACEMENT_3D('',#107210,#61172,#61173);
#50174=AXIS2_PLACEMENT_3D('',#107211,#61174,#61175);
#50175=AXIS2_PLACEMENT_3D('',#107213,#61176,#61177);
#50176=AXIS2_PLACEMENT_3D('',#107217,#61179,#61180);
#50177=AXIS2_PLACEMENT_3D('',#107221,#61182,#61183);
#50178=AXIS2_PLACEMENT_3D('',#107224,#61185,#61186);
#50179=AXIS2_PLACEMENT_3D('',#107226,#61187,#61188);
#50180=AXIS2_PLACEMENT_3D('',#107229,#61190,#61191);
#50181=AXIS2_PLACEMENT_3D('',#107230,#61192,#61193);
#50182=AXIS2_PLACEMENT_3D('',#107232,#61194,#61195);
#50183=AXIS2_PLACEMENT_3D('',#107235,#61197,#61198);
#50184=AXIS2_PLACEMENT_3D('',#107279,#61199,#61200);
#50185=AXIS2_PLACEMENT_3D('',#107281,#61201,#61202);
#50186=AXIS2_PLACEMENT_3D('',#107284,#61204,#61205);
#50187=AXIS2_PLACEMENT_3D('',#107285,#61206,#61207);
#50188=AXIS2_PLACEMENT_3D('',#107288,#61208,#61209);
#50189=AXIS2_PLACEMENT_3D('',#107292,#61211,#61212);
#50190=AXIS2_PLACEMENT_3D('',#107294,#61214,#61215);
#50191=AXIS2_PLACEMENT_3D('',#107296,#61216,#61217);
#50192=AXIS2_PLACEMENT_3D('',#107299,#61219,#61220);
#50193=AXIS2_PLACEMENT_3D('',#107300,#61221,#61222);
#50194=AXIS2_PLACEMENT_3D('',#107303,#61223,#61224);
#50195=AXIS2_PLACEMENT_3D('',#107306,#61226,#61227);
#50196=AXIS2_PLACEMENT_3D('',#107308,#61228,#61229);
#50197=AXIS2_PLACEMENT_3D('',#107319,#61230,#61231);
#50198=AXIS2_PLACEMENT_3D('',#107321,#61232,#61233);
#50199=AXIS2_PLACEMENT_3D('',#107330,#61234,#61235);
#50200=AXIS2_PLACEMENT_3D('',#107333,#61237,#61238);
#50201=AXIS2_PLACEMENT_3D('',#107334,#61239,#61240);
#50202=AXIS2_PLACEMENT_3D('',#107336,#61241,#61242);
#50203=AXIS2_PLACEMENT_3D('',#107339,#61244,#61245);
#50204=AXIS2_PLACEMENT_3D('',#107340,#61246,#61247);
#50205=AXIS2_PLACEMENT_3D('',#107343,#61248,#61249);
#50206=AXIS2_PLACEMENT_3D('',#107347,#61251,#61252);
#50207=AXIS2_PLACEMENT_3D('',#107349,#61254,#61255);
#50208=AXIS2_PLACEMENT_3D('',#107352,#61256,#61257);
#50209=AXIS2_PLACEMENT_3D('',#107356,#61259,#61260);
#50210=AXIS2_PLACEMENT_3D('',#107360,#61262,#61263);
#50211=AXIS2_PLACEMENT_3D('',#107362,#61265,#61266);
#50212=AXIS2_PLACEMENT_3D('',#107364,#61267,#61268);
#50213=AXIS2_PLACEMENT_3D('',#107367,#61270,#61271);
#50214=AXIS2_PLACEMENT_3D('',#107368,#61272,#61273);
#50215=AXIS2_PLACEMENT_3D('',#107370,#61274,#61275);
#50216=AXIS2_PLACEMENT_3D('',#107373,#61277,#61278);
#50217=AXIS2_PLACEMENT_3D('',#107374,#61279,#61280);
#50218=AXIS2_PLACEMENT_3D('',#107376,#61281,#61282);
#50219=AXIS2_PLACEMENT_3D('',#107379,#61284,#61285);
#50220=AXIS2_PLACEMENT_3D('',#107380,#61286,#61287);
#50221=AXIS2_PLACEMENT_3D('',#107382,#61288,#61289);
#50222=AXIS2_PLACEMENT_3D('',#107385,#61291,#61292);
#50223=AXIS2_PLACEMENT_3D('',#107386,#61293,#61294);
#50224=AXIS2_PLACEMENT_3D('',#107388,#61295,#61296);
#50225=AXIS2_PLACEMENT_3D('',#107392,#61298,#61299);
#50226=AXIS2_PLACEMENT_3D('',#107396,#61301,#61302);
#50227=AXIS2_PLACEMENT_3D('',#107399,#61304,#61305);
#50228=AXIS2_PLACEMENT_3D('',#107401,#61307,#61308);
#50229=AXIS2_PLACEMENT_3D('',#107403,#61309,#61310);
#50230=AXIS2_PLACEMENT_3D('',#107406,#61312,#61313);
#50231=AXIS2_PLACEMENT_3D('',#107407,#61314,#61315);
#50232=AXIS2_PLACEMENT_3D('',#107410,#61317,#61318);
#50233=AXIS2_PLACEMENT_3D('',#107414,#61320,#61321);
#50234=AXIS2_PLACEMENT_3D('',#107416,#61323,#61324);
#50235=AXIS2_PLACEMENT_3D('',#107419,#61325,#61326);
#50236=AXIS2_PLACEMENT_3D('',#107422,#61328,#61329);
#50237=AXIS2_PLACEMENT_3D('',#107424,#61330,#61331);
#50238=AXIS2_PLACEMENT_3D('',#107428,#61333,#61334);
#50239=AXIS2_PLACEMENT_3D('',#107430,#61336,#61337);
#50240=AXIS2_PLACEMENT_3D('',#107439,#61342,#61343);
#50241=AXIS2_PLACEMENT_3D('',#107444,#61345,#61346);
#50242=AXIS2_PLACEMENT_3D('',#107448,#61348,#61349);
#50243=AXIS2_PLACEMENT_3D('',#107451,#61351,#61352);
#50244=AXIS2_PLACEMENT_3D('',#107452,#61353,#61354);
#50245=AXIS2_PLACEMENT_3D('',#107453,#61355,#61356);
#50246=AXIS2_PLACEMENT_3D('',#107457,#61358,#61359);
#50247=AXIS2_PLACEMENT_3D('',#107462,#61362,#61363);
#50248=AXIS2_PLACEMENT_3D('',#107473,#61370,#61371);
#50249=AXIS2_PLACEMENT_3D('',#107482,#61377,#61378);
#50250=AXIS2_PLACEMENT_3D('',#107492,#61384,#61385);
#50251=AXIS2_PLACEMENT_3D('',#107501,#61390,#61391);
#50252=AXIS2_PLACEMENT_3D('',#107502,#61392,#61393);
#50253=AXIS2_PLACEMENT_3D('',#107506,#61395,#61396);
#50254=AXIS2_PLACEMENT_3D('',#107510,#61398,#61399);
#50255=AXIS2_PLACEMENT_3D('',#107514,#61401,#61402);
#50256=AXIS2_PLACEMENT_3D('',#107518,#61404,#61405);
#50257=AXIS2_PLACEMENT_3D('',#107519,#61406,#61407);
#50258=AXIS2_PLACEMENT_3D('',#107520,#61408,#61409);
#50259=AXIS2_PLACEMENT_3D('',#107523,#61411,#61412);
#50260=AXIS2_PLACEMENT_3D('',#107524,#61413,#61414);
#50261=AXIS2_PLACEMENT_3D('',#107525,#61415,#61416);
#50262=AXIS2_PLACEMENT_3D('',#107527,#61417,#61418);
#50263=AXIS2_PLACEMENT_3D('',#107529,#61420,#61421);
#50264=AXIS2_PLACEMENT_3D('',#107535,#61425,#61426);
#50265=AXIS2_PLACEMENT_3D('',#107548,#61433,#61434);
#50266=AXIS2_PLACEMENT_3D('',#107581,#61451,#61452);
#50267=AXIS2_PLACEMENT_3D('',#107601,#61462,#61463);
#50268=AXIS2_PLACEMENT_3D('',#107605,#61465,#61466);
#50269=AXIS2_PLACEMENT_3D('',#107609,#61468,#61469);
#50270=AXIS2_PLACEMENT_3D('',#107617,#61473,#61474);
#50271=AXIS2_PLACEMENT_3D('',#107621,#61476,#61477);
#50272=AXIS2_PLACEMENT_3D('',#107625,#61479,#61480);
#50273=AXIS2_PLACEMENT_3D('',#107630,#61483,#61484);
#50274=AXIS2_PLACEMENT_3D('',#107633,#61486,#61487);
#50275=AXIS2_PLACEMENT_3D('',#107634,#61488,#61489);
#50276=AXIS2_PLACEMENT_3D('',#107635,#61490,#61491);
#50277=AXIS2_PLACEMENT_3D('',#107641,#61495,#61496);
#50278=AXIS2_PLACEMENT_3D('',#107648,#61502,#61503);
#50279=AXIS2_PLACEMENT_3D('',#107654,#61507,#61508);
#50280=AXIS2_PLACEMENT_3D('',#107663,#61515,#61516);
#50281=AXIS2_PLACEMENT_3D('',#107669,#61520,#61521);
#50282=AXIS2_PLACEMENT_3D('',#107674,#61525,#61526);
#50283=AXIS2_PLACEMENT_3D('',#107678,#61529,#61530);
#50284=AXIS2_PLACEMENT_3D('',#107682,#61533,#61534);
#50285=AXIS2_PLACEMENT_3D('',#107684,#61536,#61537);
#50286=AXIS2_PLACEMENT_3D('',#107687,#61540,#61541);
#50287=AXIS2_PLACEMENT_3D('',#107689,#61543,#61544);
#50288=AXIS2_PLACEMENT_3D('',#107691,#61546,#61547);
#50289=AXIS2_PLACEMENT_3D('',#107693,#61549,#61550);
#50290=AXIS2_PLACEMENT_3D('',#107695,#61552,#61553);
#50291=AXIS2_PLACEMENT_3D('',#107697,#61555,#61556);
#50292=AXIS2_PLACEMENT_3D('',#107699,#61558,#61559);
#50293=AXIS2_PLACEMENT_3D('',#107700,#61560,#61561);
#50294=AXIS2_PLACEMENT_3D('',#107701,#61562,#61563);
#50295=AXIS2_PLACEMENT_3D('',#107702,#61564,#61565);
#50296=AXIS2_PLACEMENT_3D('',#107703,#61566,#61567);
#50297=AXIS2_PLACEMENT_3D('',#107708,#61571,#61572);
#50298=AXIS2_PLACEMENT_3D('',#107711,#61574,#61575);
#50299=AXIS2_PLACEMENT_3D('',#107712,#61576,#61577);
#50300=AXIS2_PLACEMENT_3D('',#107716,#61580,#61581);
#50301=AXIS2_PLACEMENT_3D('',#107719,#61583,#61584);
#50302=AXIS2_PLACEMENT_3D('',#107720,#61585,#61586);
#50303=AXIS2_PLACEMENT_3D('',#107724,#61589,#61590);
#50304=AXIS2_PLACEMENT_3D('',#107727,#61592,#61593);
#50305=AXIS2_PLACEMENT_3D('',#107728,#61594,#61595);
#50306=AXIS2_PLACEMENT_3D('',#107732,#61598,#61599);
#50307=AXIS2_PLACEMENT_3D('',#107735,#61601,#61602);
#50308=AXIS2_PLACEMENT_3D('',#107736,#61603,#61604);
#50309=AXIS2_PLACEMENT_3D('',#107739,#61607,#61608);
#50310=AXIS2_PLACEMENT_3D('',#107740,#61609,#61610);
#50311=AXIS2_PLACEMENT_3D('',#107741,#61611,#61612);
#50312=AXIS2_PLACEMENT_3D('',#107745,#61615,#61616);
#50313=AXIS2_PLACEMENT_3D('',#107747,#61617,#61618);
#50314=AXIS2_PLACEMENT_3D('',#107749,#61620,#61621);
#50315=AXIS2_PLACEMENT_3D('',#107753,#61624,#61625);
#50316=AXIS2_PLACEMENT_3D('',#107754,#61626,#61627);
#50317=AXIS2_PLACEMENT_3D('',#107755,#61628,#61629);
#50318=AXIS2_PLACEMENT_3D('',#107761,#61633,#61634);
#50319=AXIS2_PLACEMENT_3D('',#107767,#61638,#61639);
#50320=AXIS2_PLACEMENT_3D('',#107773,#61644,#61645);
#50321=AXIS2_PLACEMENT_3D('',#107775,#61647,#61648);
#50322=AXIS2_PLACEMENT_3D('',#107777,#61650,#61651);
#50323=AXIS2_PLACEMENT_3D('',#107779,#61653,#61654);
#50324=AXIS2_PLACEMENT_3D('',#107781,#61656,#61657);
#50325=AXIS2_PLACEMENT_3D('',#107783,#61659,#61660);
#50326=AXIS2_PLACEMENT_3D('',#107784,#61661,#61662);
#50327=AXIS2_PLACEMENT_3D('',#107785,#61663,#61664);
#50328=AXIS2_PLACEMENT_3D('',#107786,#61665,#61666);
#50329=AXIS2_PLACEMENT_3D('',#107787,#61667,#61668);
#50330=AXIS2_PLACEMENT_3D('',#107788,#61669,#61670);
#50331=AXIS2_PLACEMENT_3D('',#107790,#61672,#61673);
#50332=AXIS2_PLACEMENT_3D('',#107791,#61674,#61675);
#50333=AXIS2_PLACEMENT_3D('',#107792,#61676,#61677);
#50334=AXIS2_PLACEMENT_3D('',#107793,#61678,#61679);
#50335=AXIS2_PLACEMENT_3D('',#107799,#61683,#61684);
#50336=AXIS2_PLACEMENT_3D('',#107803,#61687,#61688);
#50337=AXIS2_PLACEMENT_3D('',#107807,#61691,#61692);
#50338=AXIS2_PLACEMENT_3D('',#107811,#61695,#61696);
#50339=AXIS2_PLACEMENT_3D('',#107815,#61699,#61700);
#50340=AXIS2_PLACEMENT_3D('',#107819,#61703,#61704);
#50341=AXIS2_PLACEMENT_3D('',#107823,#61707,#61708);
#50342=AXIS2_PLACEMENT_3D('',#107825,#61710,#61711);
#50343=AXIS2_PLACEMENT_3D('',#107826,#61712,#61713);
#50344=AXIS2_PLACEMENT_3D('',#107827,#61714,#61715);
#50345=AXIS2_PLACEMENT_3D('',#107828,#61716,#61717);
#50346=AXIS2_PLACEMENT_3D('',#107829,#61718,#61719);
#50347=AXIS2_PLACEMENT_3D('',#107839,#61725,#61726);
#50348=AXIS2_PLACEMENT_3D('',#107840,#61727,#61728);
#50349=AXIS2_PLACEMENT_3D('',#107841,#61729,#61730);
#50350=AXIS2_PLACEMENT_3D('',#107845,#61733,#61734);
#50351=AXIS2_PLACEMENT_3D('',#107846,#61735,#61736);
#50352=AXIS2_PLACEMENT_3D('',#107847,#61737,#61738);
#50353=AXIS2_PLACEMENT_3D('',#107849,#61740,#61741);
#50354=AXIS2_PLACEMENT_3D('',#107853,#61744,#61745);
#50355=AXIS2_PLACEMENT_3D('',#107855,#61747,#61748);
#50356=AXIS2_PLACEMENT_3D('',#107856,#61749,#61750);
#50357=AXIS2_PLACEMENT_3D('',#107858,#61752,#61753);
#50358=AXIS2_PLACEMENT_3D('',#107859,#61754,#61755);
#50359=AXIS2_PLACEMENT_3D('',#107860,#61756,#61757);
#50360=AXIS2_PLACEMENT_3D('',#107863,#61758,#61759);
#50361=AXIS2_PLACEMENT_3D('',#107866,#61762,#61763);
#50362=AXIS2_PLACEMENT_3D('',#107869,#61764,#61765);
#50363=AXIS2_PLACEMENT_3D('',#107872,#61768,#61769);
#50364=AXIS2_PLACEMENT_3D('',#107875,#61772,#61773);
#50365=AXIS2_PLACEMENT_3D('',#107876,#61774,#61775);
#61172=DIRECTION('axis',(0.,0.,1.));
#61173=DIRECTION('refdir',(1.,0.,0.));
#61174=DIRECTION('center_axis',(-1.,0.,0.));
#61175=DIRECTION('ref_axis',(0.,0.,1.));
#61176=DIRECTION('center_axis',(-1.,0.,0.));
#61177=DIRECTION('ref_axis',(0.,0.,1.));
#61178=DIRECTION('',(-1.,0.,0.));
#61179=DIRECTION('center_axis',(-1.,0.,0.));
#61180=DIRECTION('ref_axis',(0.,0.,1.));
#61181=DIRECTION('',(-1.,0.,0.));
#61182=DIRECTION('center_axis',(-1.,0.,0.));
#61183=DIRECTION('ref_axis',(0.,0.,1.));
#61184=DIRECTION('',(-1.,0.,0.));
#61185=DIRECTION('center_axis',(-1.,0.,0.));
#61186=DIRECTION('ref_axis',(0.,0.,1.));
#61187=DIRECTION('center_axis',(-1.,0.,0.));
#61188=DIRECTION('ref_axis',(0.,0.,1.));
#61189=DIRECTION('',(-1.,0.,0.));
#61190=DIRECTION('center_axis',(-1.,0.,0.));
#61191=DIRECTION('ref_axis',(0.,0.,1.));
#61192=DIRECTION('center_axis',(1.,0.,0.));
#61193=DIRECTION('ref_axis',(0.,0.,-1.));
#61194=DIRECTION('center_axis',(-1.,0.,0.));
#61195=DIRECTION('ref_axis',(0.,0.,-1.));
#61196=DIRECTION('',(1.,0.,0.));
#61197=DIRECTION('center_axis',(-1.,0.,0.));
#61198=DIRECTION('ref_axis',(0.,0.,1.));
#61199=DIRECTION('center_axis',(0.,0.,1.));
#61200=DIRECTION('ref_axis',(1.,0.,0.));
#61201=DIRECTION('center_axis',(0.,0.,-1.));
#61202=DIRECTION('ref_axis',(-1.,0.,0.));
#61203=DIRECTION('',(0.,0.,1.));
#61204=DIRECTION('center_axis',(0.,0.,1.));
#61205=DIRECTION('ref_axis',(-1.,0.,0.));
#61206=DIRECTION('center_axis',(0.,0.,1.));
#61207=DIRECTION('ref_axis',(1.,0.,0.));
#61208=DIRECTION('center_axis',(0.,0.,-1.));
#61209=DIRECTION('ref_axis',(-1.,0.,0.));
#61210=DIRECTION('',(0.,0.,-1.));
#61211=DIRECTION('center_axis',(0.,0.,-1.));
#61212=DIRECTION('ref_axis',(-1.,0.,0.));
#61213=DIRECTION('',(0.,0.,1.));
#61214=DIRECTION('center_axis',(0.,0.,-1.));
#61215=DIRECTION('ref_axis',(-1.,0.,0.));
#61216=DIRECTION('center_axis',(0.,0.,-1.));
#61217=DIRECTION('ref_axis',(-1.,0.,0.));
#61218=DIRECTION('',(0.,0.,-1.));
#61219=DIRECTION('center_axis',(0.,0.,-1.));
#61220=DIRECTION('ref_axis',(-1.,0.,0.));
#61221=DIRECTION('center_axis',(0.,0.,-1.));
#61222=DIRECTION('ref_axis',(-1.,0.,0.));
#61223=DIRECTION('center_axis',(0.,0.,1.));
#61224=DIRECTION('ref_axis',(-1.,0.,0.));
#61225=DIRECTION('',(0.64018439966448,-7.83999775913175E-17,-0.768221279597376));
#61226=DIRECTION('center_axis',(0.,0.,-1.));
#61227=DIRECTION('ref_axis',(-1.,0.,0.));
#61228=DIRECTION('center_axis',(0.,0.,1.));
#61229=DIRECTION('ref_axis',(-1.,0.,0.));
#61230=DIRECTION('center_axis',(0.,0.,-1.));
#61231=DIRECTION('ref_axis',(-1.,0.,0.));
#61232=DIRECTION('center_axis',(0.,0.,-1.));
#61233=DIRECTION('ref_axis',(-1.,0.,0.));
#61234=DIRECTION('center_axis',(0.,0.,-1.));
#61235=DIRECTION('ref_axis',(-1.,0.,0.));
#61236=DIRECTION('',(0.,0.,-1.));
#61237=DIRECTION('center_axis',(0.,0.,-1.));
#61238=DIRECTION('ref_axis',(-1.,0.,0.));
#61239=DIRECTION('center_axis',(0.,0.,1.));
#61240=DIRECTION('ref_axis',(1.,0.,0.));
#61241=DIRECTION('center_axis',(0.,0.,-1.));
#61242=DIRECTION('ref_axis',(-1.,0.,0.));
#61243=DIRECTION('',(0.,0.,1.));
#61244=DIRECTION('center_axis',(0.,0.,1.));
#61245=DIRECTION('ref_axis',(-1.,0.,0.));
#61246=DIRECTION('center_axis',(0.,0.,1.));
#61247=DIRECTION('ref_axis',(1.,0.,0.));
#61248=DIRECTION('center_axis',(0.,0.,-1.));
#61249=DIRECTION('ref_axis',(-1.,0.,0.));
#61250=DIRECTION('',(0.,0.,-1.));
#61251=DIRECTION('center_axis',(0.,0.,1.));
#61252=DIRECTION('ref_axis',(-1.,0.,0.));
#61253=DIRECTION('',(0.,0.,-1.));
#61254=DIRECTION('center_axis',(0.,0.,-1.));
#61255=DIRECTION('ref_axis',(-1.,0.,0.));
#61256=DIRECTION('center_axis',(0.,0.,1.));
#61257=DIRECTION('ref_axis',(-1.,0.,0.));
#61258=DIRECTION('',(0.,0.,-1.));
#61259=DIRECTION('center_axis',(0.,0.,1.));
#61260=DIRECTION('ref_axis',(-1.,0.,0.));
#61261=DIRECTION('',(0.,0.,-1.));
#61262=DIRECTION('center_axis',(0.,0.,1.));
#61263=DIRECTION('ref_axis',(-1.,0.,0.));
#61264=DIRECTION('',(0.,0.,-1.));
#61265=DIRECTION('center_axis',(0.,0.,1.));
#61266=DIRECTION('ref_axis',(1.,0.,0.));
#61267=DIRECTION('center_axis',(0.,0.,1.));
#61268=DIRECTION('ref_axis',(1.,0.,0.));
#61269=DIRECTION('',(0.,0.,1.));
#61270=DIRECTION('center_axis',(0.,0.,1.));
#61271=DIRECTION('ref_axis',(1.,0.,0.));
#61272=DIRECTION('center_axis',(0.,0.,1.));
#61273=DIRECTION('ref_axis',(1.,0.,0.));
#61274=DIRECTION('center_axis',(0.,0.,1.));
#61275=DIRECTION('ref_axis',(1.,0.,0.));
#61276=DIRECTION('',(0.,0.,1.));
#61277=DIRECTION('center_axis',(0.,0.,1.));
#61278=DIRECTION('ref_axis',(1.,0.,0.));
#61279=DIRECTION('center_axis',(0.,0.,1.));
#61280=DIRECTION('ref_axis',(1.,0.,0.));
#61281=DIRECTION('center_axis',(0.,0.,1.));
#61282=DIRECTION('ref_axis',(1.,0.,0.));
#61283=DIRECTION('',(0.,0.,1.));
#61284=DIRECTION('center_axis',(0.,0.,1.));
#61285=DIRECTION('ref_axis',(1.,0.,0.));
#61286=DIRECTION('center_axis',(0.,0.,-1.));
#61287=DIRECTION('ref_axis',(-1.,0.,0.));
#61288=DIRECTION('center_axis',(0.,0.,1.));
#61289=DIRECTION('ref_axis',(1.,0.,0.));
#61290=DIRECTION('',(0.,0.,-1.));
#61291=DIRECTION('center_axis',(0.,0.,1.));
#61292=DIRECTION('ref_axis',(1.,0.,0.));
#61293=DIRECTION('center_axis',(0.,0.,-1.));
#61294=DIRECTION('ref_axis',(-1.,0.,0.));
#61295=DIRECTION('center_axis',(0.,0.,1.));
#61296=DIRECTION('ref_axis',(1.,0.,0.));
#61297=DIRECTION('',(0.,0.,-1.));
#61298=DIRECTION('center_axis',(0.,0.,-1.));
#61299=DIRECTION('ref_axis',(-1.,0.,0.));
#61300=DIRECTION('',(0.,0.,1.));
#61301=DIRECTION('center_axis',(0.,0.,-1.));
#61302=DIRECTION('ref_axis',(-1.,0.,0.));
#61303=DIRECTION('',(0.,0.,-1.));
#61304=DIRECTION('center_axis',(0.,0.,1.));
#61305=DIRECTION('ref_axis',(1.,0.,0.));
#61306=DIRECTION('',(0.,0.,1.));
#61307=DIRECTION('center_axis',(0.,0.,-1.));
#61308=DIRECTION('ref_axis',(-1.,0.,0.));
#61309=DIRECTION('center_axis',(0.,0.,1.));
#61310=DIRECTION('ref_axis',(1.,0.,0.));
#61311=DIRECTION('',(0.,0.,-1.));
#61312=DIRECTION('center_axis',(0.,0.,1.));
#61313=DIRECTION('ref_axis',(1.,0.,0.));
#61314=DIRECTION('center_axis',(0.,0.,1.));
#61315=DIRECTION('ref_axis',(1.,0.,0.));
#61316=DIRECTION('',(0.,0.,1.));
#61317=DIRECTION('center_axis',(0.,0.,-1.));
#61318=DIRECTION('ref_axis',(-1.,0.,0.));
#61319=DIRECTION('',(0.,0.,1.));
#61320=DIRECTION('center_axis',(0.,0.,-1.));
#61321=DIRECTION('ref_axis',(-1.,0.,0.));
#61322=DIRECTION('',(0.,0.,-1.));
#61323=DIRECTION('center_axis',(0.,0.,-1.));
#61324=DIRECTION('ref_axis',(-1.,0.,0.));
#61325=DIRECTION('center_axis',(0.,0.,1.));
#61326=DIRECTION('ref_axis',(1.,0.,0.));
#61327=DIRECTION('',(0.,0.,-1.));
#61328=DIRECTION('center_axis',(0.,0.,-1.));
#61329=DIRECTION('ref_axis',(-1.,0.,0.));
#61330=DIRECTION('center_axis',(0.,0.,-1.));
#61331=DIRECTION('ref_axis',(-1.,0.,0.));
#61332=DIRECTION('',(0.,0.,1.));
#61333=DIRECTION('center_axis',(0.,0.,1.));
#61334=DIRECTION('ref_axis',(1.,0.,0.));
#61335=DIRECTION('',(0.,0.,-1.));
#61336=DIRECTION('center_axis',(-4.08908562752743E-48,1.,2.5571182003049E-32));
#61337=DIRECTION('ref_axis',(1.,8.50802870020078E-63,1.59909918401107E-16));
#61338=DIRECTION('',(1.01043442692316E-14,1.E-14,1.));
#61339=DIRECTION('',(0.984628016341329,1.01574517857485E-14,0.17466444811621));
#61340=DIRECTION('',(0.,0.,1.));
#61341=DIRECTION('',(-0.984628016341329,-1.01574517857485E-14,0.174664448116209));
#61342=DIRECTION('center_axis',(0.,0.,1.));
#61343=DIRECTION('ref_axis',(1.,0.,0.));
#61344=DIRECTION('',(0.,0.,1.));
#61345=DIRECTION('center_axis',(0.,0.,1.));
#61346=DIRECTION('ref_axis',(-1.,0.,0.));
#61347=DIRECTION('',(0.,0.,-1.));
#61348=DIRECTION('center_axis',(0.,0.,1.));
#61349=DIRECTION('ref_axis',(-1.,0.,0.));
#61350=DIRECTION('',(0.,0.,1.));
#61351=DIRECTION('center_axis',(0.,0.,1.));
#61352=DIRECTION('ref_axis',(-1.,0.,0.));
#61353=DIRECTION('center_axis',(0.,0.,1.));
#61354=DIRECTION('ref_axis',(-1.,0.,0.));
#61355=DIRECTION('center_axis',(0.,0.,1.));
#61356=DIRECTION('ref_axis',(1.,0.,0.));
#61357=DIRECTION('',(1.,-1.00901155052454E-14,0.));
#61358=DIRECTION('center_axis',(0.,0.,1.));
#61359=DIRECTION('ref_axis',(-1.,0.,0.));
#61360=DIRECTION('',(0.,-1.,0.));
#61361=DIRECTION('',(0.,1.,0.));
#61362=DIRECTION('center_axis',(0.,0.,1.));
#61363=DIRECTION('ref_axis',(-1.,0.,0.));
#61364=DIRECTION('',(1.0838294844996E-14,1.,0.));
#61365=DIRECTION('',(0.707106781186546,-0.707106781186549,0.));
#61366=DIRECTION('',(0.225189398770639,-0.97431500793189,0.));
#61367=DIRECTION('',(0.,-1.,0.));
#61368=DIRECTION('',(-0.707106781186549,0.707106781186546,0.));
#61369=DIRECTION('',(0.,-1.,0.));
#61370=DIRECTION('center_axis',(0.,0.,-1.));
#61371=DIRECTION('ref_axis',(0.,-1.,0.));
#61372=DIRECTION('',(-0.707106781186551,-0.707106781186544,0.));
#61373=DIRECTION('',(1.,1.0159909918401E-14,0.));
#61374=DIRECTION('',(1.0159909918401E-14,-1.,0.));
#61375=DIRECTION('',(0.,-1.,0.));
#61376=DIRECTION('',(1.,-1.00901155052454E-14,0.));
#61377=DIRECTION('center_axis',(1.60527967783421E-47,7.69222732429044E-32,
1.));
#61378=DIRECTION('ref_axis',(1.,-2.08688538463375E-16,-3.50729211666941E-63));
#61379=DIRECTION('',(-0.707106781186551,-0.707106781186544,0.));
#61380=DIRECTION('',(1.,-1.00901155052454E-14,0.));
#61381=DIRECTION('',(0.,-1.,0.));
#61382=DIRECTION('',(1.0159909918401E-14,-1.,0.));
#61383=DIRECTION('',(-1.,-1.0159909918401E-14,1.02086885384633E-14));
#61384=DIRECTION('center_axis',(-0.707106781186549,0.707106781186546,0.));
#61385=DIRECTION('ref_axis',(0.,0.,1.));
#61386=DIRECTION('',(0.,0.,-1.));
#61387=DIRECTION('',(0.701608823197059,0.701608823197062,-0.124459304288878));
#61388=DIRECTION('',(0.,0.,-1.));
#61389=DIRECTION('',(-0.707106781186546,-0.707106781186549,0.));
#61390=DIRECTION('center_axis',(0.,0.,-1.));
#61391=DIRECTION('ref_axis',(0.,-1.,0.));
#61392=DIRECTION('center_axis',(0.,0.,1.));
#61393=DIRECTION('ref_axis',(-1.,-6.4252467419967E-13,0.));
#61394=DIRECTION('',(-1.10484358065218E-14,-1.,0.));
#61395=DIRECTION('center_axis',(0.,0.,1.));
#61396=DIRECTION('ref_axis',(-1.,0.,0.));
#61397=DIRECTION('',(0.640406508926595,-0.768036134126807,0.));
#61398=DIRECTION('center_axis',(0.,0.,-1.));
#61399=DIRECTION('ref_axis',(-1.,0.,0.));
#61400=DIRECTION('',(-1.15041237245925E-14,-1.,0.));
#61401=DIRECTION('center_axis',(0.,0.,1.));
#61402=DIRECTION('ref_axis',(1.,0.,0.));
#61403=DIRECTION('',(0.707106781186548,-0.707106781186547,0.));
#61404=DIRECTION('center_axis',(0.,0.,1.));
#61405=DIRECTION('ref_axis',(-1.,0.,0.));
#61406=DIRECTION('center_axis',(0.,0.,-1.));
#61407=DIRECTION('ref_axis',(-1.,0.,0.));
#61408=DIRECTION('center_axis',(0.,0.,-1.));
#61409=DIRECTION('ref_axis',(-1.,0.,0.));
#61410=DIRECTION('',(0.,0.,-1.));
#61411=DIRECTION('center_axis',(0.,0.,1.));
#61412=DIRECTION('ref_axis',(-1.,0.,0.));
#61413=DIRECTION('center_axis',(0.,0.,-1.));
#61414=DIRECTION('ref_axis',(-1.,0.,0.));
#61415=DIRECTION('center_axis',(0.,0.,1.));
#61416=DIRECTION('ref_axis',(1.,0.,0.));
#61417=DIRECTION('center_axis',(0.,0.,1.));
#61418=DIRECTION('ref_axis',(-1.,0.,0.));
#61419=DIRECTION('',(0.,0.,1.));
#61420=DIRECTION('center_axis',(0.,-1.,0.));
#61421=DIRECTION('ref_axis',(0.,0.,-1.));
#61422=DIRECTION('',(-1.,0.,0.));
#61423=DIRECTION('',(0.,0.,-1.));
#61424=DIRECTION('',(-1.,0.,0.));
#61425=DIRECTION('center_axis',(0.,-1.,0.));
#61426=DIRECTION('ref_axis',(0.,0.,-1.));
#61427=DIRECTION('',(-1.,0.,0.));
#61428=DIRECTION('',(0.,0.,-1.));
#61429=DIRECTION('',(-1.,0.,0.));
#61430=DIRECTION('',(0.,0.,-1.));
#61431=DIRECTION('',(-1.,1.0031973271849E-14,0.));
#61432=DIRECTION('',(0.,0.,1.));
#61433=DIRECTION('center_axis',(0.,0.,-1.));
#61434=DIRECTION('ref_axis',(0.,-1.,0.));
#61435=DIRECTION('',(0.,1.,0.));
#61436=DIRECTION('',(-0.707106781186547,0.707106781186548,0.));
#61437=DIRECTION('',(-1.,0.,0.));
#61438=DIRECTION('',(-0.707106781186548,-0.707106781186548,0.));
#61439=DIRECTION('',(-1.0000695223269E-14,-1.,0.));
#61440=DIRECTION('',(0.707106781186547,-0.707106781186548,0.));
#61441=DIRECTION('',(1.,1.0159909918401E-14,0.));
#61442=DIRECTION('',(0.707106781186546,0.707106781186549,0.));
#61443=DIRECTION('',(0.,-1.,0.));
#61444=DIRECTION('',(-0.309086072337564,-0.951034068730946,0.));
#61445=DIRECTION('',(-1.,0.,0.));
#61446=DIRECTION('',(-0.309086072337565,0.951034068730946,0.));
#61447=DIRECTION('',(0.,1.,0.));
#61448=DIRECTION('',(0.309086072337565,0.951034068730946,0.));
#61449=DIRECTION('',(1.,0.,0.));
#61450=DIRECTION('',(0.309086072337564,-0.951034068730946,0.));
#61451=DIRECTION('center_axis',(0.,0.,-1.));
#61452=DIRECTION('ref_axis',(0.,-1.,0.));
#61453=DIRECTION('',(-0.707106781186547,-0.707106781186548,0.));
#61454=DIRECTION('',(1.0159909918401E-14,-1.,0.));
#61455=DIRECTION('',(1.,1.0159909918401E-14,0.));
#61456=DIRECTION('',(0.707106781186547,-0.707106781186548,0.));
#61457=DIRECTION('',(-1.0000695223269E-14,-1.,0.));
#61458=DIRECTION('',(-0.707106781186548,-0.707106781186548,0.));
#61459=DIRECTION('',(-1.,0.,0.));
#61460=DIRECTION('',(-0.707106781186547,0.707106781186548,0.));
#61461=DIRECTION('',(1.0838294844996E-14,1.,0.));
#61462=DIRECTION('center_axis',(0.,0.,-1.));
#61463=DIRECTION('ref_axis',(1.,0.,0.));
#61464=DIRECTION('',(-0.640406508926594,0.768036134126808,0.));
#61465=DIRECTION('center_axis',(0.,0.,1.));
#61466=DIRECTION('ref_axis',(-1.,0.,0.));
#61467=DIRECTION('',(-1.15041237245925E-14,1.,0.));
#61468=DIRECTION('center_axis',(0.,0.,-1.));
#61469=DIRECTION('ref_axis',(-1.,0.,0.));
#61470=DIRECTION('',(-0.707106781186549,0.707106781186546,0.));
#61471=DIRECTION('',(1.0159909918401E-14,-1.,0.));
#61472=DIRECTION('',(0.707106781186548,-0.707106781186547,0.));
#61473=DIRECTION('center_axis',(0.,0.,1.));
#61474=DIRECTION('ref_axis',(1.,0.,0.));
#61475=DIRECTION('',(-1.15041237245925E-14,-1.,0.));
#61476=DIRECTION('center_axis',(0.,0.,-1.));
#61477=DIRECTION('ref_axis',(-1.,0.,0.));
#61478=DIRECTION('',(0.640406508926595,-0.768036134126807,0.));
#61479=DIRECTION('center_axis',(0.,0.,1.));
#61480=DIRECTION('ref_axis',(-1.,0.,0.));
#61481=DIRECTION('',(-1.10484358065218E-14,-1.,0.));
#61482=DIRECTION('',(1.,0.,0.));
#61483=DIRECTION('center_axis',(0.,0.,1.));
#61484=DIRECTION('ref_axis',(-1.,0.,0.));
#61485=DIRECTION('',(1.01439313087194E-14,1.,0.));
#61486=DIRECTION('center_axis',(0.,0.,1.));
#61487=DIRECTION('ref_axis',(-1.,0.,0.));
#61488=DIRECTION('center_axis',(0.,0.,-1.));
#61489=DIRECTION('ref_axis',(-1.,0.,0.));
#61490=DIRECTION('center_axis',(0.707106781186548,0.707106781186548,0.));
#61491=DIRECTION('ref_axis',(0.,0.,-1.));
#61492=DIRECTION('',(0.,0.,-1.));
#61493=DIRECTION('',(-0.707106781186547,0.707106781186548,0.));
#61494=DIRECTION('',(0.,0.,-1.));
#61495=DIRECTION('center_axis',(-4.08908562752742E-48,1.,2.55711820030489E-32));
#61496=DIRECTION('ref_axis',(1.,1.39774757217584E-62,1.59909918401107E-16));
#61497=DIRECTION('',(-0.984628016341329,-1.01574517857485E-14,0.174664448116209));
#61498=DIRECTION('',(-1.,-1.0159909918401E-14,0.));
#61499=DIRECTION('',(0.,0.,-1.));
#61500=DIRECTION('',(0.984628016341329,1.01574517857485E-14,0.17466444811621));
#61501=DIRECTION('',(0.,0.,-1.));
#61502=DIRECTION('center_axis',(-0.707106781186549,0.707106781186546,0.));
#61503=DIRECTION('ref_axis',(0.,0.,1.));
#61504=DIRECTION('',(0.,0.,-1.));
#61505=DIRECTION('',(-0.701608823197059,-0.701608823197062,-0.124459304288878));
#61506=DIRECTION('',(0.577350269189623,0.577350269189625,0.577350269189629));
#61507=DIRECTION('center_axis',(-1.,0.,0.));
#61508=DIRECTION('ref_axis',(0.,0.,1.));
#61509=DIRECTION('',(1.0159909918401E-14,-1.,0.));
#61510=DIRECTION('',(1.0159909918401E-14,-1.,0.));
#61511=DIRECTION('',(1.0159909918401E-14,-1.,0.));
#61512=DIRECTION('',(0.,0.,-1.));
#61513=DIRECTION('',(0.,0.,-1.));
#61514=DIRECTION('',(0.,-1.,0.));
#61515=DIRECTION('center_axis',(-0.974315007931891,-0.225189398770632,0.));
#61516=DIRECTION('ref_axis',(-0.225189398770632,0.974315007931891,0.));
#61517=DIRECTION('',(0.,0.,-1.));
#61518=DIRECTION('',(0.1989949751698,-0.860980986979965,0.468094798001619));
#61519=DIRECTION('',(0.219688060005901,-0.950512657770367,-0.219688060005904));
#61520=DIRECTION('center_axis',(-0.707106781186549,-0.707106781186547,0.));
#61521=DIRECTION('ref_axis',(-0.707106781186547,0.707106781186549,0.));
#61522=DIRECTION('',(0.,0.,-1.));
#61523=DIRECTION('',(0.,0.,-1.));
#61524=DIRECTION('',(0.707106781186547,-0.707106781186548,0.));
#61525=DIRECTION('center_axis',(0.,-1.,0.));
#61526=DIRECTION('ref_axis',(0.,0.,-1.));
#61527=DIRECTION('',(0.,0.,-1.));
#61528=DIRECTION('',(1.,0.,0.));
#61529=DIRECTION('center_axis',(0.707106781186548,-0.707106781186548,0.));
#61530=DIRECTION('ref_axis',(0.,0.,-1.));
#61531=DIRECTION('',(0.,0.,-1.));
#61532=DIRECTION('',(0.707106781186548,0.707106781186548,0.));
#61533=DIRECTION('center_axis',(1.,-6.95223269150415E-19,0.));
#61534=DIRECTION('ref_axis',(0.,0.,1.));
#61535=DIRECTION('',(1.0000695223269E-14,1.,0.));
#61536=DIRECTION('center_axis',(0.500000000000001,0.500000000000001,-0.707106781186546));
#61537=DIRECTION('ref_axis',(-1.20310517779348E-15,-0.816496580927725,-0.577350269189628));
#61538=DIRECTION('',(0.678598344545843,0.281084637714825,0.67859834454585));
#61539=DIRECTION('',(-0.281084637714825,-0.678598344545842,-0.67859834454585));
#61540=DIRECTION('center_axis',(-1.13073387680411E-16,0.707106781186552,
-0.707106781186544));
#61541=DIRECTION('ref_axis',(-1.,1.02474602976116E-31,1.59909918401109E-16));
#61542=DIRECTION('',(0.28108463771482,-0.678598344545843,-0.678598344545851));
#61543=DIRECTION('center_axis',(0.707106781186552,-4.91597088054941E-19,
-0.707106781186544));
#61544=DIRECTION('ref_axis',(4.41380838164238E-34,-1.,6.95223269150422E-19));
#61545=DIRECTION('',(0.678598344545842,-0.281084637714827,0.67859834454585));
#61546=DIRECTION('center_axis',(-0.500000000000002,0.500000000000002,-0.707106781186545));
#61547=DIRECTION('ref_axis',(-0.816496580927723,2.47688303890596E-15,0.57735026918963));
#61548=DIRECTION('',(0.678598344545844,-0.281084637714819,-0.678598344545851));
#61549=DIRECTION('center_axis',(0.500000000000001,-0.500000000000001,-0.707106781186546));
#61550=DIRECTION('ref_axis',(8.28813430912774E-16,-0.816496580927725,0.577350269189628));
#61551=DIRECTION('',(0.281084637714827,-0.678598344545842,0.67859834454585));
#61552=DIRECTION('center_axis',(-0.707106781186552,0.,-0.707106781186544));
#61553=DIRECTION('ref_axis',(-0.707106781186544,0.,0.707106781186552));
#61554=DIRECTION('',(0.678598344545843,0.281084637714824,-0.67859834454585));
#61555=DIRECTION('center_axis',(0.,-0.707106781186552,-0.707106781186544));
#61556=DIRECTION('ref_axis',(0.,0.707106781186544,-0.707106781186552));
#61557=DIRECTION('',(-0.281084637714825,-0.678598344545843,0.67859834454585));
#61558=DIRECTION('center_axis',(-0.500000000000001,-0.500000000000001,-0.707106781186546));
#61559=DIRECTION('ref_axis',(-0.816496580927724,-1.85046612426036E-15,0.577350269189628));
#61560=DIRECTION('center_axis',(0.,0.,1.));
#61561=DIRECTION('ref_axis',(1.,0.,0.));
#61562=DIRECTION('center_axis',(0.,0.,1.));
#61563=DIRECTION('ref_axis',(1.,0.,0.));
#61564=DIRECTION('center_axis',(0.,0.,1.));
#61565=DIRECTION('ref_axis',(1.,0.,0.));
#61566=DIRECTION('center_axis',(-0.707106781186546,-0.707106781186549,0.));
#61567=DIRECTION('ref_axis',(-0.707106781186549,0.707106781186546,0.));
#61568=DIRECTION('',(-0.577350269189625,0.577350269189622,-0.577350269189631));
#61569=DIRECTION('',(0.,0.,-1.));
#61570=DIRECTION('',(0.707106781186549,-0.707106781186546,0.));
#61571=DIRECTION('center_axis',(0.,0.,-1.));
#61572=DIRECTION('ref_axis',(-1.,0.,0.));
#61573=DIRECTION('',(0.,0.,-1.));
#61574=DIRECTION('center_axis',(0.,0.,1.));
#61575=DIRECTION('ref_axis',(-1.,-3.33694734056382E-12,0.));
#61576=DIRECTION('center_axis',(-1.,-1.50412372459265E-15,0.));
#61577=DIRECTION('ref_axis',(-1.50412372459265E-15,1.,0.));
#61578=DIRECTION('',(0.,0.,-1.));
#61579=DIRECTION('',(1.15041237245925E-14,-1.,0.));
#61580=DIRECTION('center_axis',(0.,0.,-1.));
#61581=DIRECTION('ref_axis',(-1.,0.,0.));
#61582=DIRECTION('',(0.,0.,-1.));
#61583=DIRECTION('center_axis',(0.,0.,-1.));
#61584=DIRECTION('ref_axis',(-1.,0.,0.));
#61585=DIRECTION('center_axis',(-0.768036134126809,-0.640406508926593,0.));
#61586=DIRECTION('ref_axis',(-0.640406508926593,0.768036134126809,0.));
#61587=DIRECTION('',(0.,0.,-1.));
#61588=DIRECTION('',(0.640406508926594,-0.768036134126808,0.));
#61589=DIRECTION('center_axis',(0.,0.,-1.));
#61590=DIRECTION('ref_axis',(-1.,0.,0.));
#61591=DIRECTION('',(0.,0.,-1.));
#61592=DIRECTION('center_axis',(0.,0.,1.));
#61593=DIRECTION('ref_axis',(-1.,0.,0.));
#61594=DIRECTION('center_axis',(-1.,8.38294844996084E-16,0.));
#61595=DIRECTION('ref_axis',(0.,0.,1.));
#61596=DIRECTION('',(0.,0.,-1.));
#61597=DIRECTION('',(-1.0838294844996E-14,-1.,0.));
#61598=DIRECTION('center_axis',(0.,0.,1.));
#61599=DIRECTION('ref_axis',(1.,0.,0.));
#61600=DIRECTION('',(0.,0.,1.));
#61601=DIRECTION('center_axis',(0.,0.,1.));
#61602=DIRECTION('ref_axis',(-1.,0.,0.));
#61603=DIRECTION('center_axis',(0.,0.,-1.));
#61604=DIRECTION('ref_axis',(0.,-1.,0.));
#61605=DIRECTION('',(0.,1.,0.));
#61606=DIRECTION('',(0.,-1.,0.));
#61607=DIRECTION('center_axis',(1.,0.,0.));
#61608=DIRECTION('ref_axis',(0.,1.,0.));
#61609=DIRECTION('center_axis',(-1.,0.,0.));
#61610=DIRECTION('ref_axis',(0.,0.,1.));
#61611=DIRECTION('center_axis',(0.,1.,0.));
#61612=DIRECTION('ref_axis',(1.,0.,0.));
#61613=DIRECTION('',(1.,0.,0.));
#61614=DIRECTION('',(0.,0.,-1.));
#61615=DIRECTION('center_axis',(0.,0.,-1.));
#61616=DIRECTION('ref_axis',(0.707106781186543,-0.707106781186553,0.));
#61617=DIRECTION('center_axis',(0.,0.,1.));
#61618=DIRECTION('ref_axis',(-1.,0.,0.));
#61619=DIRECTION('',(0.,0.,-1.));
#61620=DIRECTION('center_axis',(-1.,1.43931308719534E-16,0.));
#61621=DIRECTION('ref_axis',(0.,0.,1.));
#61622=DIRECTION('',(1.02398855145324E-14,1.,0.));
#61623=DIRECTION('',(0.,0.,-1.));
#61624=DIRECTION('center_axis',(0.,0.,-1.));
#61625=DIRECTION('ref_axis',(0.707106781186539,0.707106781186556,0.));
#61626=DIRECTION('center_axis',(0.,0.,1.));
#61627=DIRECTION('ref_axis',(1.,0.,0.));
#61628=DIRECTION('center_axis',(0.707106781186548,-0.707106781186547,0.));
#61629=DIRECTION('ref_axis',(0.,0.,-1.));
#61630=DIRECTION('',(0.,0.,-1.));
#61631=DIRECTION('',(-0.577350269189624,-0.577350269189624,-0.57735026918963));
#61632=DIRECTION('',(-0.707106781186547,-0.707106781186548,0.));
#61633=DIRECTION('center_axis',(1.,0.,0.));
#61634=DIRECTION('ref_axis',(0.,1.,0.));
#61635=DIRECTION('',(0.,0.,-1.));
#61636=DIRECTION('',(0.,-1.,-1.0159909918401E-14));
#61637=DIRECTION('',(0.,-1.,0.));
#61638=DIRECTION('center_axis',(0.707106781186547,0.707106781186548,0.));
#61639=DIRECTION('ref_axis',(0.,0.,-1.));
#61640=DIRECTION('',(0.577350269189624,-0.577350269189624,0.57735026918963));
#61641=DIRECTION('',(0.707106781186548,-0.707106781186547,0.));
#61642=DIRECTION('',(0.,0.,-1.));
#61643=DIRECTION('',(0.,0.,-1.));
#61644=DIRECTION('center_axis',(0.,0.,-1.));
#61645=DIRECTION('ref_axis',(-1.,0.,0.));
#61646=DIRECTION('',(0.,0.,-1.));
#61647=DIRECTION('center_axis',(1.,-1.50412372459265E-15,0.));
#61648=DIRECTION('ref_axis',(0.,0.,1.));
#61649=DIRECTION('',(0.,0.,-1.));
#61650=DIRECTION('center_axis',(0.,0.,-1.));
#61651=DIRECTION('ref_axis',(-1.,0.,0.));
#61652=DIRECTION('',(0.,0.,-1.));
#61653=DIRECTION('center_axis',(0.768036134126808,0.640406508926594,0.));
#61654=DIRECTION('ref_axis',(0.,0.,-1.));
#61655=DIRECTION('',(0.,0.,-1.));
#61656=DIRECTION('center_axis',(0.,0.,-1.));
#61657=DIRECTION('ref_axis',(-1.,0.,0.));
#61658=DIRECTION('',(0.,0.,-1.));
#61659=DIRECTION('center_axis',(1.,-1.0484358065219E-15,0.));
#61660=DIRECTION('ref_axis',(0.,0.,1.));
#61661=DIRECTION('center_axis',(-0.707106781186551,-1.13073387680411E-16,
0.707106781186544));
#61662=DIRECTION('ref_axis',(-1.59909918401107E-16,1.,2.60143314432367E-31));
#61663=DIRECTION('center_axis',(0.,0.,1.));
#61664=DIRECTION('ref_axis',(-0.914066015001456,-0.405565432722463,0.));
#61665=DIRECTION('center_axis',(0.,0.,1.));
#61666=DIRECTION('ref_axis',(-1.,0.,0.));
#61667=DIRECTION('center_axis',(0.,0.,-1.));
#61668=DIRECTION('ref_axis',(0.,-1.,0.));
#61669=DIRECTION('center_axis',(0.,0.,1.));
#61670=DIRECTION('ref_axis',(1.,0.,0.));
#61671=DIRECTION('',(0.766044443118981,0.642787609686536,0.));
#61672=DIRECTION('center_axis',(0.,0.,-1.));
#61673=DIRECTION('ref_axis',(0.,-1.,0.));
#61674=DIRECTION('center_axis',(0.,0.,-1.));
#61675=DIRECTION('ref_axis',(0.,-1.,0.));
#61676=DIRECTION('center_axis',(0.,0.,-1.));
#61677=DIRECTION('ref_axis',(0.,-1.,0.));
#61678=DIRECTION('center_axis',(-0.951034068730948,0.309086072337558,0.));
#61679=DIRECTION('ref_axis',(0.,0.,1.));
#61680=DIRECTION('',(0.,0.,1.));
#61681=DIRECTION('',(-0.309086072337564,-0.951034068730946,0.));
#61682=DIRECTION('',(0.,0.,1.));
#61683=DIRECTION('center_axis',(0.,1.,0.));
#61684=DIRECTION('ref_axis',(1.,0.,0.));
#61685=DIRECTION('',(-1.,0.,0.));
#61686=DIRECTION('',(0.,0.,1.));
#61687=DIRECTION('center_axis',(0.951034068730948,0.309086072337558,0.));
#61688=DIRECTION('ref_axis',(0.,0.,-1.));
#61689=DIRECTION('',(-0.309086072337565,0.951034068730946,0.));
#61690=DIRECTION('',(0.,0.,1.));
#61691=DIRECTION('center_axis',(1.,0.,0.));
#61692=DIRECTION('ref_axis',(0.,1.,0.));
#61693=DIRECTION('',(0.,1.,0.));
#61694=DIRECTION('',(0.,0.,1.));
#61695=DIRECTION('center_axis',(0.951034068730948,-0.309086072337558,0.));
#61696=DIRECTION('ref_axis',(0.,0.,-1.));
#61697=DIRECTION('',(0.309086072337565,0.951034068730946,0.));
#61698=DIRECTION('',(0.,0.,1.));
#61699=DIRECTION('center_axis',(0.,-1.,0.));
#61700=DIRECTION('ref_axis',(0.,0.,-1.));
#61701=DIRECTION('',(1.,0.,0.));
#61702=DIRECTION('',(0.,0.,1.));
#61703=DIRECTION('center_axis',(-0.951034068730948,-0.309086072337558,0.));
#61704=DIRECTION('ref_axis',(-0.309086072337558,0.951034068730948,0.));
#61705=DIRECTION('',(0.309086072337564,-0.951034068730946,0.));
#61706=DIRECTION('',(0.,0.,1.));
#61707=DIRECTION('center_axis',(-1.,0.,0.));
#61708=DIRECTION('ref_axis',(0.,0.,1.));
#61709=DIRECTION('',(0.,-1.,0.));
#61710=DIRECTION('center_axis',(0.,0.,-1.));
#61711=DIRECTION('ref_axis',(0.,-1.,0.));
#61712=DIRECTION('center_axis',(0.,0.,-1.));
#61713=DIRECTION('ref_axis',(-1.,0.,0.));
#61714=DIRECTION('center_axis',(0.,0.,1.));
#61715=DIRECTION('ref_axis',(-1.,0.,0.));
#61716=DIRECTION('center_axis',(0.,0.,-1.));
#61717=DIRECTION('ref_axis',(0.,-1.,0.));
#61718=DIRECTION('center_axis',(0.642787609686535,-0.766044443118982,0.));
#61719=DIRECTION('ref_axis',(0.,0.,-1.));
#61720=DIRECTION('',(-0.766044443118981,-0.642787609686536,0.));
#61721=DIRECTION('',(0.,0.,-1.));
#61722=DIRECTION('',(0.766044443118981,0.642787609686536,0.));
#61723=DIRECTION('',(0.,0.,1.));
#61724=DIRECTION('',(-0.766044443118981,-0.642787609686536,0.));
#61725=DIRECTION('center_axis',(0.,0.,-1.));
#61726=DIRECTION('ref_axis',(-1.,0.,0.));
#61727=DIRECTION('center_axis',(0.,0.,1.));
#61728=DIRECTION('ref_axis',(1.,0.,0.));
#61729=DIRECTION('center_axis',(0.,0.,-1.));
#61730=DIRECTION('ref_axis',(0.,-1.,0.));
#61731=DIRECTION('',(-1.0159909918401E-14,1.,0.));
#61732=DIRECTION('',(1.,1.0159909918401E-14,0.));
#61733=DIRECTION('center_axis',(0.174664448116201,2.79305776458362E-17,
0.98462801634133));
#61734=DIRECTION('ref_axis',(1.59909918401107E-16,-1.,1.11324494830527E-31));
#61735=DIRECTION('center_axis',(0.174664448116202,2.79305776458363E-17,
-0.98462801634133));
#61736=DIRECTION('ref_axis',(1.74870334563606E-32,-1.,-2.8366629003327E-17));
#61737=DIRECTION('center_axis',(-0.707106781186544,0.707106781186551,7.37825403516808E-17));
#61738=DIRECTION('ref_axis',(1.04344269231688E-16,3.03340043204828E-31,
1.));
#61739=DIRECTION('',(1.01043442692316E-14,1.E-14,1.));
#61740=DIRECTION('center_axis',(0.,0.,-1.));
#61741=DIRECTION('ref_axis',(0.,-1.,0.));
#61742=DIRECTION('',(0.,1.,0.));
#61743=DIRECTION('',(1.,1.13010426069825E-14,0.));
#61744=DIRECTION('center_axis',(1.,0.,-1.04344269231688E-16));
#61745=DIRECTION('ref_axis',(0.,1.,0.));
#61746=DIRECTION('',(1.01043442692316E-14,1.E-14,1.));
#61747=DIRECTION('center_axis',(1.30104260698259E-15,-1.,-1.19070656486426E-31));
#61748=DIRECTION('ref_axis',(1.04509199371491E-63,1.19070656486426E-31,
-1.));
#61749=DIRECTION('center_axis',(-9.01155052455486E-17,-1.,2.60887201197534E-32));
#61750=DIRECTION('ref_axis',(-1.,9.01155052455486E-17,0.));
#61751=DIRECTION('',(1.01043442692316E-14,1.E-14,1.));
#61752=DIRECTION('center_axis',(-1.,0.,1.04344269231688E-16));
#61753=DIRECTION('ref_axis',(0.,1.,0.));
#61754=DIRECTION('center_axis',(1.,0.,0.));
#61755=DIRECTION('ref_axis',(0.,1.,0.));
#61756=DIRECTION('center_axis',(1.,0.,0.));
#61757=DIRECTION('ref_axis',(0.,1.,0.));
#61758=DIRECTION('center_axis',(-1.,0.,0.));
#61759=DIRECTION('ref_axis',(0.,0.,1.));
#61760=DIRECTION('',(0.,0.,-1.));
#61761=DIRECTION('',(0.,0.,1.));
#61762=DIRECTION('center_axis',(-1.,0.,0.));
#61763=DIRECTION('ref_axis',(0.,1.89882151931499E-15,-1.));
#61764=DIRECTION('center_axis',(-1.,0.,0.));
#61765=DIRECTION('ref_axis',(0.,0.,1.));
#61766=DIRECTION('',(1.,0.,0.));
#61767=DIRECTION('',(-1.,0.,0.));
#61768=DIRECTION('center_axis',(-1.,0.,0.));
#61769=DIRECTION('ref_axis',(0.,0.,1.));
#61770=DIRECTION('',(0.,0.,1.));
#61771=DIRECTION('',(0.,0.,-1.));
#61772=DIRECTION('center_axis',(0.,1.,0.));
#61773=DIRECTION('ref_axis',(1.,0.,0.));
#61774=DIRECTION('center_axis',(0.,-1.,0.));
#61775=DIRECTION('ref_axis',(0.,0.,-1.));
#107210=CARTESIAN_POINT('',(0.,0.,0.));
#107211=CARTESIAN_POINT('Origin',(-0.0411262178068916,-0.00152418147196182,
0.079));
#107212=CARTESIAN_POINT('',(-0.0286262178069016,-0.00152418147196182,0.071));
#107213=CARTESIAN_POINT('Origin',(-0.0286262178069016,-0.00152418147197183,
0.07900000000001));
#107214=CARTESIAN_POINT('',(-0.0321262178069016,-0.00152418147196182,0.071));
#107215=CARTESIAN_POINT('',(-0.0411262178068916,-0.00152418147196182,0.071));
#107216=CARTESIAN_POINT('',(-0.0321262178068916,-0.00552418147196183,0.0859282032302755));
#107217=CARTESIAN_POINT('Origin',(-0.0321262178069016,-0.00152418147197183,
0.07900000000001));
#107218=CARTESIAN_POINT('',(-0.0381262178068916,-0.00552418147196183,0.0859282032302755));
#107219=CARTESIAN_POINT('',(0.0161247821931184,-0.00552418147197183,0.0859282032302855));
#107220=CARTESIAN_POINT('',(-0.0381262178069016,-0.00152418147196182,0.071));
#107221=CARTESIAN_POINT('Origin',(-0.0381262178069016,-0.00152418147197183,
0.07900000000001));
#107222=CARTESIAN_POINT('',(-0.0411262178069016,-0.00152418147196182,0.071));
#107223=CARTESIAN_POINT('',(-0.0411262178068916,-0.00152418147196182,0.071));
#107224=CARTESIAN_POINT('Origin',(-0.0411262178069016,-0.00152418147197183,
0.07900000000001));
#107225=CARTESIAN_POINT('',(-0.0381262178068916,0.00247581852803818,0.0859282032302755));
#107226=CARTESIAN_POINT('Origin',(-0.0381262178069016,-0.00152418147197183,
0.07900000000001));
#107227=CARTESIAN_POINT('',(-0.0321262178068916,0.00247581852803818,0.0859282032302755));
#107228=CARTESIAN_POINT('',(0.0161247821931184,0.00247581852804817,0.0859282032302855));
#107229=CARTESIAN_POINT('Origin',(-0.0321262178069016,-0.00152418147197183,
0.07900000000001));
#107230=CARTESIAN_POINT('Origin',(-0.0411262178068916,-0.00152418147196182,
0.079));
#107231=CARTESIAN_POINT('',(-0.0286262178069016,-0.00152418147196182,0.081125));
#107232=CARTESIAN_POINT('Origin',(-0.0286262178069016,-0.00152418147197183,
0.07900000000001));
#107233=CARTESIAN_POINT('',(0.0121237821931184,-0.00152418147197183,0.08112500000002));
#107234=CARTESIAN_POINT('',(-0.0411262178068916,-0.00152418147196182,0.081125));
#107235=CARTESIAN_POINT('Origin',(0.0121237821931184,-0.00152418147197183,
0.07900000000001));
#107236=CARTESIAN_POINT('',(-0.0203797546539288,-0.000224178970103186,0.0773190423874585));
#107237=CARTESIAN_POINT('Ctrl Pts',(-0.0203762178068916,-0.00022418147196183,
0.0773190404525986));
#107238=CARTESIAN_POINT('Ctrl Pts',(-0.0206041367243007,-0.00022418147196183,
0.0773190404525986));
#107239=CARTESIAN_POINT('Ctrl Pts',(-0.0208484971135947,-0.000190393504626254,
0.0773434259833289));
#107240=CARTESIAN_POINT('Ctrl Pts',(-0.0212999007338416,-5.9145278846161E-5,
0.0774582802029004));
#107241=CARTESIAN_POINT('Ctrl Pts',(-0.0215066409493357,3.78043950968824E-5,
0.0775505157144276));
#107242=CARTESIAN_POINT('Ctrl Pts',(-0.0218058691331723,0.000218825249262259,
0.0777773576396814));
#107243=CARTESIAN_POINT('Ctrl Pts',(-0.0219377558664678,0.000320335511817705,
0.0779313118315859));
#107244=CARTESIAN_POINT('Ctrl Pts',(-0.0220899352670536,0.000453326551835115,
0.0782097791064571));
#107245=CARTESIAN_POINT('Ctrl Pts',(-0.0221452961494637,0.000508622809583374,
0.078359759662944));
#107246=CARTESIAN_POINT('Ctrl Pts',(-0.0222161284923853,0.000582494315132349,
0.0786773256153168));
#107247=CARTESIAN_POINT('Ctrl Pts',(-0.0222321205521884,0.00060081852803818,
0.0788448530223251));
#107248=CARTESIAN_POINT('Ctrl Pts',(-0.0222321205521884,0.00060081852803818,
0.0791551469776749));
#107249=CARTESIAN_POINT('Ctrl Pts',(-0.0222161284923853,0.000582494315132348,
0.0793226743846832));
#107250=CARTESIAN_POINT('Ctrl Pts',(-0.0221452961494636,0.000508622809583367,
0.079640240337056));
#107251=CARTESIAN_POINT('Ctrl Pts',(-0.0220899352670536,0.000453326551835114,
0.0797902208935429));
#107252=CARTESIAN_POINT('Ctrl Pts',(-0.0219377558664678,0.000320335511817702,
0.0800686881684141));
#107253=CARTESIAN_POINT('Ctrl Pts',(-0.0218058691331723,0.000218825249262255,
0.0802226423603186));
#107254=CARTESIAN_POINT('Ctrl Pts',(-0.0215066409493357,3.78043950968792E-5,
0.0804494842855724));
#107255=CARTESIAN_POINT('Ctrl Pts',(-0.0212999007338416,-5.91452788461605E-5,
0.0805417197970996));
#107256=CARTESIAN_POINT('Ctrl Pts',(-0.0208484971135947,-0.000190393504626253,
0.0806565740166711));
#107257=CARTESIAN_POINT('Ctrl Pts',(-0.0206041367243007,-0.00022418147196183,
0.0806809595474014));
#107258=CARTESIAN_POINT('Ctrl Pts',(-0.0201482988894825,-0.00022418147196183,
0.0806809595474014));
#107259=CARTESIAN_POINT('Ctrl Pts',(-0.0199039385001885,-0.000190393504626255,
0.0806565740166711));
#107260=CARTESIAN_POINT('Ctrl Pts',(-0.0194525348799416,-5.91452788461642E-5,
0.0805417197970996));
#107261=CARTESIAN_POINT('Ctrl Pts',(-0.0192457946644475,3.78043950968792E-5,
0.0804494842855724));
#107262=CARTESIAN_POINT('Ctrl Pts',(-0.0189465664806109,0.000218825249262255,
0.0802226423603186));
#107263=CARTESIAN_POINT('Ctrl Pts',(-0.0188146797473154,0.000320335511817702,
0.0800686881684141));
#107264=CARTESIAN_POINT('Ctrl Pts',(-0.0186625003467296,0.000453326551835114,
0.0797902208935429));
#107265=CARTESIAN_POINT('Ctrl Pts',(-0.0186071394643196,0.000508622809583367,
0.079640240337056));
#107266=CARTESIAN_POINT('Ctrl Pts',(-0.0185363071213979,0.000582494315132348,
0.0793226743846832));
#107267=CARTESIAN_POINT('Ctrl Pts',(-0.0185203150615948,0.00060081852803818,
0.0791551469776749));
#107268=CARTESIAN_POINT('Ctrl Pts',(-0.0185203150615948,0.00060081852803818,
0.0788448530223251));
#107269=CARTESIAN_POINT('Ctrl Pts',(-0.0185363071213979,0.000582494315132347,
0.0786773256153168));
#107270=CARTESIAN_POINT('Ctrl Pts',(-0.0186071394643196,0.000508622809583367,
0.078359759662944));
#107271=CARTESIAN_POINT('Ctrl Pts',(-0.0186625003467296,0.000453326551835115,
0.0782097791064571));
#107272=CARTESIAN_POINT('Ctrl Pts',(-0.0188146797473154,0.000320335511817705,
0.0779313118315859));
#107273=CARTESIAN_POINT('Ctrl Pts',(-0.0189465664806109,0.000218825249262259,
0.0777773576396814));
#107274=CARTESIAN_POINT('Ctrl Pts',(-0.0192457946644475,3.78043950968827E-5,
0.0775505157144276));
#107275=CARTESIAN_POINT('Ctrl Pts',(-0.0194525348799416,-5.91452788461609E-5,
0.0774582802029004));
#107276=CARTESIAN_POINT('Ctrl Pts',(-0.0199039385001885,-0.000190393504626253,
0.0773434259833289));
#107277=CARTESIAN_POINT('Ctrl Pts',(-0.0201482988894825,-0.00022418147196183,
0.0773190404525986));
#107278=CARTESIAN_POINT('Ctrl Pts',(-0.0203762178068916,-0.00022418147196183,
0.0773190404525986));
#107279=CARTESIAN_POINT('Origin',(-0.00312621780689159,0.00227581852803817,
0.041107864376269));
#107280=CARTESIAN_POINT('',(-0.00612621780691159,0.00227581852804816,0.05525000000001));
#107281=CARTESIAN_POINT('Origin',(-0.0031262178069016,0.00227581852804816,
0.05525000000001));
#107282=CARTESIAN_POINT('',(-0.00612621780691159,0.00227581852804816,0.05660000000001));
#107283=CARTESIAN_POINT('',(-0.00612621780689159,0.00227581852803817,0.041107864376269));
#107284=CARTESIAN_POINT('Origin',(-0.0031262178069016,0.00227581852804816,
0.05660000000001));
#107285=CARTESIAN_POINT('Origin',(-0.00312621780689159,0.00227581852803817,
0.041107864376269));
#107286=CARTESIAN_POINT('',(-0.00719324679239884,0.00518430184946944,0.05525));
#107287=CARTESIAN_POINT('',(-0.00719324679239884,-0.000632664793393113,
0.05525));
#107288=CARTESIAN_POINT('Origin',(-0.0031262178069016,0.00227581852804816,
0.05525000000001));
#107289=CARTESIAN_POINT('',(-0.00719324679239884,0.00518430184946944,0.0566));
#107290=CARTESIAN_POINT('',(-0.00719324679240884,0.00518430184947944,0.05592500000001));
#107291=CARTESIAN_POINT('',(-0.00719324679239884,-0.000632664793393113,
0.0566));
#107292=CARTESIAN_POINT('Origin',(-0.0031262178069016,0.00227581852804816,
0.05660000000001));
#107293=CARTESIAN_POINT('',(-0.00719324679240884,-0.000632664793403113,
0.05592500000001));
#107294=CARTESIAN_POINT('Origin',(-0.0203762178068916,0.00227581852803817,
0.0862));
#107295=CARTESIAN_POINT('',(-0.0178762178068916,0.00227581852803817,0.08620000000001));
#107296=CARTESIAN_POINT('Origin',(-0.0203762178069016,0.00227581852804817,
0.08620000000001));
#107297=CARTESIAN_POINT('',(-0.0178762178068916,0.00227581852803817,0.07370000000001));
#107298=CARTESIAN_POINT('',(-0.0178762178068916,0.00227581852803817,0.0862));
#107299=CARTESIAN_POINT('Origin',(-0.0203762178069016,0.00227581852804817,
0.07370000000001));
#107300=CARTESIAN_POINT('Origin',(-0.0203762178068916,0.00227581852803817,
0.0637));
#107301=CARTESIAN_POINT('',(-0.0144609098358771,-0.00594152633560559,0.0586));
#107302=CARTESIAN_POINT('',(-0.0102512178068916,0.00227581852803817,0.05860000000001));
#107303=CARTESIAN_POINT('Origin',(-0.0203762178069016,0.00227581852804817,
0.05860000000001));
#107304=CARTESIAN_POINT('',(-0.00912621780688617,0.00227581852803817,0.0572499999999935));
#107305=CARTESIAN_POINT('',(-0.0145012178068916,0.00227581852803817,0.0637));
#107306=CARTESIAN_POINT('Origin',(-0.0203762178069016,0.00227581852804817,
0.05725000000001));
#107307=CARTESIAN_POINT('',(-0.0144609098358771,0.0104931633916819,0.0586));
#107308=CARTESIAN_POINT('Origin',(-0.0203762178069016,0.00227581852804817,
0.05860000000001));
#107309=CARTESIAN_POINT('',(-0.0164233917199351,0.0066559059616719,0.06367));
#107310=CARTESIAN_POINT('Ctrl Pts',(-0.0164233917199351,0.0066559059616719,
0.06367));
#107311=CARTESIAN_POINT('Ctrl Pts',(-0.0164194276971006,0.00666794003675013,
0.0636560923266654));
#107312=CARTESIAN_POINT('Ctrl Pts',(-0.0164154450144916,0.00667997579433552,
0.0636421601590875));
#107313=CARTESIAN_POINT('Ctrl Pts',(-0.0159684806507079,0.00802457625950158,
0.0620832010103005));
#107314=CARTESIAN_POINT('Ctrl Pts',(-0.0153003449699402,0.00932716537760438,
0.0603240800152843));
#107315=CARTESIAN_POINT('Ctrl Pts',(-0.0144793567578685,0.0104676731934383,
0.0586377577447297));
#107316=CARTESIAN_POINT('Ctrl Pts',(-0.0144701478215295,0.0104804208666844,
0.058618886548445));
#107317=CARTESIAN_POINT('Ctrl Pts',(-0.0144609098358771,0.0104931633916819,
0.0586));
#107318=CARTESIAN_POINT('',(-0.0262762178068916,0.00227581852803817,0.06367));
#107319=CARTESIAN_POINT('Origin',(-0.0203762178069016,0.00227581852804817,
0.06367000000001));
#107320=CARTESIAN_POINT('',(-0.0164233917199351,-0.00210426890559556,0.06367));
#107321=CARTESIAN_POINT('Origin',(-0.0203762178069016,0.00227581852804817,
0.06367000000001));
#107322=CARTESIAN_POINT('Ctrl Pts',(-0.0144609098358771,-0.00594152633560559,
0.0586));
#107323=CARTESIAN_POINT('Ctrl Pts',(-0.0144701478215295,-0.00592878381060804,
0.058618886548445));
#107324=CARTESIAN_POINT('Ctrl Pts',(-0.0144793567578685,-0.00591603613736201,
0.0586377577447297));
#107325=CARTESIAN_POINT('Ctrl Pts',(-0.0153003449699402,-0.00477552832152804,
0.0603240800152843));
#107326=CARTESIAN_POINT('Ctrl Pts',(-0.0159684806507079,-0.00347293920342524,
0.0620832010103005));
#107327=CARTESIAN_POINT('Ctrl Pts',(-0.0164154450144916,-0.00212833873825919,
0.0636421601590875));
#107328=CARTESIAN_POINT('Ctrl Pts',(-0.0164194276971006,-0.00211630298067379,
0.0636560923266654));
#107329=CARTESIAN_POINT('Ctrl Pts',(-0.0164233917199351,-0.00210426890559556,
0.06367));
#107330=CARTESIAN_POINT('Origin',(-0.0203762178068916,0.00227581852803817,
0.05725));
#107331=CARTESIAN_POINT('',(-0.0091262178068916,0.00227581852803817,0.05525000000001));
#107332=CARTESIAN_POINT('',(-0.0091262178068916,0.00227581852803817,0.05725));
#107333=CARTESIAN_POINT('Origin',(-0.0203762178069016,0.00227581852804817,
0.05525000000001));
#107334=CARTESIAN_POINT('Origin',(-0.0186262178068916,-0.0128741814719618,
0.0450676623509137));
#107335=CARTESIAN_POINT('',(-0.0201262178069116,-0.0128741814719718,0.05525000000001));
#107336=CARTESIAN_POINT('Origin',(-0.0186262178069016,-0.0128741814719718,
0.05525000000001));
#107337=CARTESIAN_POINT('',(-0.0201262178069116,-0.0128741814719718,0.05660000000001));
#107338=CARTESIAN_POINT('',(-0.0201262178068916,-0.0128741814719618,0.0450676623509137));
#107339=CARTESIAN_POINT('Origin',(-0.0186262178069016,-0.0128741814719718,
0.05660000000001));
#107340=CARTESIAN_POINT('Origin',(-0.0186262178068916,-0.0128741814719618,
0.0450676623509137));
#107341=CARTESIAN_POINT('',(-0.0159420398647638,-0.0104751840199009,0.05525));
#107342=CARTESIAN_POINT('',(-0.017783602829574,-0.0163741814719618,0.05525));
#107343=CARTESIAN_POINT('Origin',(-0.0186262178069016,-0.0128741814719718,
0.05525000000001));
#107344=CARTESIAN_POINT('',(-0.0159420398647638,-0.0104751840199009,0.06075));
#107345=CARTESIAN_POINT('',(-0.0159420398647739,-0.0104751840199109,0.05592500000001));
#107346=CARTESIAN_POINT('',(-0.017783602829574,-0.0163741814719618,0.06075));
#107347=CARTESIAN_POINT('Origin',(-0.0186262178069016,-0.0128741814719718,
0.06075000000001));
#107348=CARTESIAN_POINT('',(-0.017783602829584,-0.0163741814719718,0.0450676623509237));
#107349=CARTESIAN_POINT('Origin',(-0.00487621780689159,0.0177758185280382,
0.0566));
#107350=CARTESIAN_POINT('',(-0.00681722270126977,0.0209258185280382,0.0655));
#107351=CARTESIAN_POINT('',(-0.0084892273106359,0.0169782206808412,0.0655));
#107352=CARTESIAN_POINT('Origin',(-0.00487621780690159,0.0177758185280482,
0.06550000000001));
#107353=CARTESIAN_POINT('',(-0.00681722270126977,0.0209258185280382,0.05525));
#107354=CARTESIAN_POINT('',(-0.00681722270127977,0.0209258185280481,0.05660000000001));
#107355=CARTESIAN_POINT('',(-0.00122621780689159,0.0171696007453891,0.05525));
#107356=CARTESIAN_POINT('Origin',(-0.00487621780690159,0.0177758185280482,
0.05525000000001));
#107357=CARTESIAN_POINT('',(-0.00122621780689159,0.0171696007453891,0.0566));
#107358=CARTESIAN_POINT('',(-0.00122621780690159,0.0171696007453991,0.05660000000001));
#107359=CARTESIAN_POINT('',(-0.0084892273106359,0.0169782206808412,0.0566));
#107360=CARTESIAN_POINT('Origin',(-0.00487621780690159,0.0177758185280482,
0.05660000000001));
#107361=CARTESIAN_POINT('',(-0.0084892273106459,0.0169782206808512,0.06550000000001));
#107362=CARTESIAN_POINT('Origin',(-0.0358762178068916,0.0177758185280382,
0.08545));
#107363=CARTESIAN_POINT('',(-0.0387012178068916,0.0177758185280382,0.08545000000001));
#107364=CARTESIAN_POINT('Origin',(-0.0358762178069016,0.0177758185280482,
0.08545000000001));
#107365=CARTESIAN_POINT('',(-0.0387012178068916,0.0177758185280382,0.08925000000001));
#107366=CARTESIAN_POINT('',(-0.0387012178068916,0.0177758185280382,0.08545));
#107367=CARTESIAN_POINT('Origin',(-0.0358762178069016,0.0177758185280482,
0.08925000000001));
#107368=CARTESIAN_POINT('Origin',(-0.00487621780689159,0.0177758185280382,
0.08545));
#107369=CARTESIAN_POINT('',(-0.00770121780689159,0.0177758185280382,0.08545000000001));
#107370=CARTESIAN_POINT('Origin',(-0.00487621780690159,0.0177758185280482,
0.08545000000001));
#107371=CARTESIAN_POINT('',(-0.00770121780689159,0.0177758185280382,0.08925000000001));
#107372=CARTESIAN_POINT('',(-0.00770121780689159,0.0177758185280382,0.08545));
#107373=CARTESIAN_POINT('Origin',(-0.00487621780690159,0.0177758185280482,
0.08925000000001));
#107374=CARTESIAN_POINT('Origin',(-0.0358762178068916,-0.0132241814719618,
0.08545));
#107375=CARTESIAN_POINT('',(-0.0387012178068916,-0.0132241814719618,0.08545000000001));
#107376=CARTESIAN_POINT('Origin',(-0.0358762178069016,-0.0132241814719718,
0.08545000000001));
#107377=CARTESIAN_POINT('',(-0.0387012178068916,-0.0132241814719618,0.08925000000001));
#107378=CARTESIAN_POINT('',(-0.0387012178068916,-0.0132241814719618,0.08545));
#107379=CARTESIAN_POINT('Origin',(-0.0358762178069016,-0.0132241814719718,
0.08925000000001));
#107380=CARTESIAN_POINT('Origin',(-0.0358762178068916,-0.0132241814719618,
0.08925));
#107381=CARTESIAN_POINT('',(-0.0342762178068916,-0.0132241814719718,0.08545000000001));
#107382=CARTESIAN_POINT('Origin',(-0.0358762178069016,-0.0132241814719718,
0.08545000000001));
#107383=CARTESIAN_POINT('',(-0.0342762178068916,-0.0132241814719718,0.05525000000001));
#107384=CARTESIAN_POINT('',(-0.0342762178068916,-0.0132241814719618,0.08925));
#107385=CARTESIAN_POINT('Origin',(-0.0358762178069016,-0.0132241814719718,
0.05525000000001));
#107386=CARTESIAN_POINT('Origin',(-0.00487621780689159,0.0177758185280382,
0.08925));
#107387=CARTESIAN_POINT('',(-0.00327621780689159,0.0177758185280482,0.08545000000001));
#107388=CARTESIAN_POINT('Origin',(-0.00487621780690159,0.0177758185280482,
0.08545000000001));
#107389=CARTESIAN_POINT('',(-0.00327621780689159,0.0177758185280382,0.0677));
#107390=CARTESIAN_POINT('',(-0.00327621780689159,0.0177758185280382,0.08925));
#107391=CARTESIAN_POINT('',(-0.00647621780689159,0.0177758185280382,0.0677));
#107392=CARTESIAN_POINT('Origin',(-0.00487621780690159,0.0177758185280482,
0.06770000000001));
#107393=CARTESIAN_POINT('',(-0.00647621780689159,0.0177758185280382,0.0586));
#107394=CARTESIAN_POINT('',(-0.00647621780690159,0.0177758185280482,0.05860000000001));
#107395=CARTESIAN_POINT('',(-0.00327621780689159,0.0177758185280382,0.0586));
#107396=CARTESIAN_POINT('Origin',(-0.00487621780690159,0.0177758185280482,
0.05860000000001));
#107397=CARTESIAN_POINT('',(-0.00327621780689159,0.0177758185280482,0.05525000000001));
#107398=CARTESIAN_POINT('',(-0.00327621780689159,0.0177758185280382,0.08925));
#107399=CARTESIAN_POINT('Origin',(-0.00487621780690159,0.0177758185280482,
0.05525000000001));
#107400=CARTESIAN_POINT('',(-0.0032762178069016,0.0177758185280482,0.05860000000001));
#107401=CARTESIAN_POINT('Origin',(-0.0358762178068916,0.0177758185280382,
0.08925));
#107402=CARTESIAN_POINT('',(-0.0342762178068916,0.0177758185280482,0.08545000000001));
#107403=CARTESIAN_POINT('Origin',(-0.0358762178069016,0.0177758185280482,
0.08545000000001));
#107404=CARTESIAN_POINT('',(-0.0342762178068916,0.0177758185280482,0.05525000000001));
#107405=CARTESIAN_POINT('',(-0.0342762178068916,0.0177758185280382,0.08925));
#107406=CARTESIAN_POINT('Origin',(-0.0358762178069016,0.0177758185280482,
0.05525000000001));
#107407=CARTESIAN_POINT('Origin',(-0.0203762178068916,0.00227581852803817,
0.05525));
#107408=CARTESIAN_POINT('',(-0.0262762178069116,0.00227581852804817,0.07370000000001));
#107409=CARTESIAN_POINT('',(-0.0262762178068916,0.00227581852803817,0.05525));
#107410=CARTESIAN_POINT('Origin',(-0.0203762178069016,0.00227581852804817,
0.07370000000001));
#107411=CARTESIAN_POINT('',(-0.0164233917199351,0.0066559059616719,0.0677));
#107412=CARTESIAN_POINT('',(-0.0164233917199451,0.0066559059616819,0.06147500000001));
#107413=CARTESIAN_POINT('',(-0.0164233917199351,-0.00210426890559556,0.0677));
#107414=CARTESIAN_POINT('Origin',(-0.0203762178069016,0.00227581852804817,
0.06770000000001));
#107415=CARTESIAN_POINT('',(-0.0164233917199451,-0.00210426890560557,0.06147500000001));
#107416=CARTESIAN_POINT('Origin',(-0.0203762178068916,0.00227581852803817,
0.0566));
#107417=CARTESIAN_POINT('',(-0.0135678120097901,0.0139332457957502,0.0655));
#107418=CARTESIAN_POINT('',(-0.0256278910009942,-0.0101608180213808,0.0655));
#107419=CARTESIAN_POINT('Origin',(-0.0203762178069016,0.00227581852804817,
0.06550000000001));
#107420=CARTESIAN_POINT('',(-0.0135678120097901,0.0139332457957502,0.0566));
#107421=CARTESIAN_POINT('',(-0.0135678120098001,0.0139332457957602,0.06550000000001));
#107422=CARTESIAN_POINT('Origin',(-0.0203762178069016,0.00227581852804817,
0.05660000000001));
#107423=CARTESIAN_POINT('',(-0.0217866356183144,-0.0111503023412681,0.05525));
#107424=CARTESIAN_POINT('Origin',(-0.0203762178069016,0.00227581852804817,
0.05525000000001));
#107425=CARTESIAN_POINT('',(-0.0217866356183144,-0.0111503023412681,0.0615));
#107426=CARTESIAN_POINT('',(-0.0217866356183244,-0.0111503023412781,0.05592500000001));
#107427=CARTESIAN_POINT('',(-0.0256278910009942,-0.0101608180213808,0.0615));
#107428=CARTESIAN_POINT('Origin',(-0.0203762178069016,0.00227581852804817,
0.06150000000001));
#107429=CARTESIAN_POINT('',(-0.0256278910010042,-0.0101608180213908,0.06550000000001));
#107430=CARTESIAN_POINT('Origin',(-0.0411262178068916,-0.0144741814719618,
0.05525));
#107431=CARTESIAN_POINT('',(0.0021237821931084,-0.0144741814719618,0.06355));
#107432=CARTESIAN_POINT('',(0.00212378219310841,-0.0144741814719618,0.08475));
#107433=CARTESIAN_POINT('',(0.0021237821931184,-0.0144741814719718,0.0326378260227564));
#107434=CARTESIAN_POINT('',(0.0121237821931084,-0.0144741814719618,0.0653239130434783));
#107435=CARTESIAN_POINT('',(0.0021237821931184,-0.0144741814719718,0.06355000000001));
#107436=CARTESIAN_POINT('',(0.0121237821931084,-0.0144741814719618,0.0829760869565217));
#107437=CARTESIAN_POINT('',(0.0121237821931184,-0.0144741814719718,0.0653239130434883));
#107438=CARTESIAN_POINT('',(0.0121237821931184,-0.0144741814719718,0.0829760869565317));
#107439=CARTESIAN_POINT('Origin',(-0.0031262178068916,0.00227581852803817,
0.0586));
#107440=CARTESIAN_POINT('',(-0.0153915143789277,-0.00447418147196182,0.06355));
#107441=CARTESIAN_POINT('',(-0.0153915143789277,-0.00447418147196182,0.0677));
#107442=CARTESIAN_POINT('',(-0.0153915143789377,-0.00447418147197182,0.05860000000001));
#107443=CARTESIAN_POINT('',(0.0021237821931084,-0.0107025288243792,0.06355));
#107444=CARTESIAN_POINT('Origin',(-0.00312621780690161,0.00227581852804816,
0.06355000000001));
#107445=CARTESIAN_POINT('',(0.00212378219310841,-0.0107025288243792,0.0677));
#107446=CARTESIAN_POINT('',(0.0021237821931184,-0.0107025288243892,0.05860000000001));
#107447=CARTESIAN_POINT('',(0.00744576188789692,-0.00690204861705493,0.0677));
#107448=CARTESIAN_POINT('Origin',(-0.00312621780690161,0.00227581852804816,
0.06770000000001));
#107449=CARTESIAN_POINT('',(0.00744576188789692,-0.00690204861705493,0.0586));
#107450=CARTESIAN_POINT('',(0.00744576188790692,-0.00690204861706493,0.05860000000001));
#107451=CARTESIAN_POINT('Origin',(-0.00312621780690161,0.00227581852804816,
0.05860000000001));
#107452=CARTESIAN_POINT('Origin',(-0.00312621780690161,0.00227581852804816,
0.06770000000001));
#107453=CARTESIAN_POINT('Origin',(-0.0411262178068916,-0.0184741814719619,
0.0677));
#107454=CARTESIAN_POINT('',(0.00212378219310841,-0.00447418147196182,0.0677));
#107455=CARTESIAN_POINT('',(-0.0411262178069016,-0.00447418147197182,0.06770000000001));
#107456=CARTESIAN_POINT('',(-0.00647621780689159,0.0158691073133175,0.0677));
#107457=CARTESIAN_POINT('Origin',(-0.00312621780690161,0.00227581852804816,
0.06770000000001));
#107458=CARTESIAN_POINT('',(-0.00647621780690159,0.0177758185280482,0.06770000000001));
#107459=CARTESIAN_POINT('',(-0.00327621780689159,0.0162750149335466,0.0677));
#107460=CARTESIAN_POINT('',(-0.0032762178069016,0.0177758185280482,0.06770000000001));
#107461=CARTESIAN_POINT('',(0.000873782193108408,0.0156922263930369,0.0677));
#107462=CARTESIAN_POINT('Origin',(-0.00312621780690161,0.00227581852804816,
0.06770000000001));
#107463=CARTESIAN_POINT('',(0.000873782193108408,0.0185258185280382,0.0677));
#107464=CARTESIAN_POINT('',(0.000873782193118408,0.0185258185280481,0.06770000000001));
#107465=CARTESIAN_POINT('',(0.0112230245980259,0.00817657612312065,0.0677));
#107466=CARTESIAN_POINT('',(0.000873782193118408,0.0185258185280481,0.06770000000001));
#107467=CARTESIAN_POINT('',(0.0121237821931084,0.00427931609139309,0.0677));
#107468=CARTESIAN_POINT('',(0.0112230245980359,0.00817657612313065,0.06770000000001));
#107469=CARTESIAN_POINT('',(0.0121237821931084,-0.0115800689222664,0.0677));
#107470=CARTESIAN_POINT('',(0.0121237821931184,0.00427931609140309,0.06770000000001));
#107471=CARTESIAN_POINT('',(0.00500246184955876,-0.00445874857871678,0.06770000000001));
#107472=CARTESIAN_POINT('',(0.00212378219311841,-0.0184741814719718,0.06770000000001));
#107473=CARTESIAN_POINT('Origin',(-0.0311262178068916,-0.0144741814719618,
0.06355));
#107474=CARTESIAN_POINT('',(-0.0171262178068915,-0.00447418147196182,0.06355));
#107475=CARTESIAN_POINT('',(-0.0311262178068916,-0.0184741814719619,0.06355));
#107476=CARTESIAN_POINT('',(-0.0311262178069016,-0.0184741814719718,0.06355000000001));
#107477=CARTESIAN_POINT('',(0.0021237821931084,-0.0184741814719618,0.06355));
#107478=CARTESIAN_POINT('',(-0.0311262178069016,-0.0184741814719718,0.06355000000001));
#107479=CARTESIAN_POINT('',(0.0021237821931184,-0.0144741814719718,0.06355000000001));
#107480=CARTESIAN_POINT('',(0.0021237821931184,-0.00447418147197182,0.06355000000001));
#107481=CARTESIAN_POINT('',(-0.0171262178069015,-0.00447418147197182,0.06355000000001));
#107482=CARTESIAN_POINT('Origin',(-0.0311262178068916,-0.0144741814719618,
0.08475));
#107483=CARTESIAN_POINT('',(-0.0171262178068915,-0.00447418147196182,0.08475));
#107484=CARTESIAN_POINT('',(-0.0311262178068916,-0.0184741814719619,0.08475));
#107485=CARTESIAN_POINT('',(-0.0311262178069016,-0.0184741814719718,0.08475000000001));
#107486=CARTESIAN_POINT('',(0.00212378219310841,-0.00447418147196182,0.08475));
#107487=CARTESIAN_POINT('',(-0.0171262178069015,-0.00447418147197182,0.08475000000001));
#107488=CARTESIAN_POINT('',(0.00212378219311841,-0.00447418147197182,0.08475000000001));
#107489=CARTESIAN_POINT('',(0.0021237821931084,-0.0184741814719618,0.08475));
#107490=CARTESIAN_POINT('',(0.0021237821931184,-0.0144741814719718,0.08475000000001));
#107491=CARTESIAN_POINT('',(-0.0311262178069016,-0.0184741814719718,0.08475000000001));
#107492=CARTESIAN_POINT('Origin',(0.0121237821931084,-0.0150800689222664,
0.08925));
#107493=CARTESIAN_POINT('',(0.00872966964341299,-0.0184741814719619,0.088));
#107494=CARTESIAN_POINT('',(0.00872966964341299,-0.0184741814719618,0.0835781730088155));
#107495=CARTESIAN_POINT('',(0.00872966964342298,-0.0184741814719718,0.08925000000001));
#107496=CARTESIAN_POINT('',(0.0121237821931084,-0.0150800689222664,0.0829760869565217));
#107497=CARTESIAN_POINT('',(0.0115759331517965,-0.0156279179635983,0.0830732706125575));
#107498=CARTESIAN_POINT('',(0.0121237821931084,-0.0150800689222664,0.088));
#107499=CARTESIAN_POINT('',(0.0121237821931184,-0.0150800689222764,0.08925000000001));
#107500=CARTESIAN_POINT('',(0.0121237821931184,-0.0150800689222764,0.08800000000001));
#107501=CARTESIAN_POINT('Origin',(-0.00487621780689159,0.0177758185280382,
0.0566));
#107502=CARTESIAN_POINT('Origin',(-0.0031262178069016,0.00227581852804816,
0.05660000000001));
#107503=CARTESIAN_POINT('',(-0.0012262178068916,0.0105512709814273,0.0566));
#107504=CARTESIAN_POINT('',(-0.0012262178069016,0.0105512709814373,0.05660000000001));
#107505=CARTESIAN_POINT('',(0.000282704463412254,0.00638543403208472,0.0566));
#107506=CARTESIAN_POINT('Origin',(0.00527877065166022,0.0105512709814373,
0.05660000000001));
#107507=CARTESIAN_POINT('',(0.000905971897274149,0.00563795269990278,0.0566));
#107508=CARTESIAN_POINT('',(0.000905971897284156,0.00563795269991278,0.05660000000001));
#107509=CARTESIAN_POINT('',(0.0021237821931084,0.00227581852803816,0.0566));
#107510=CARTESIAN_POINT('Origin',(-0.0031262178069016,0.00227581852804816,
0.05660000000001));
#107511=CARTESIAN_POINT('',(0.0021237821931084,-0.00233742823514713,0.0566));
#107512=CARTESIAN_POINT('',(0.0021237821931184,0.00227581852804816,0.05660000000001));
#107513=CARTESIAN_POINT('',(0.00358824828717567,-0.00587296214107986,0.0566));
#107514=CARTESIAN_POINT('Origin',(0.00712378219311841,-0.00233742823515713,
0.05660000000001));
#107515=CARTESIAN_POINT('',(0.00719958354106424,-0.00948429739496843,0.0566));
#107516=CARTESIAN_POINT('',(0.0100237821931184,-0.0123084960470226,0.05660000000001));
#107517=CARTESIAN_POINT('',(-0.0135678120097901,-0.00938160873967384,0.0566));
#107518=CARTESIAN_POINT('Origin',(-0.0031262178069016,0.00227581852804816,
0.05660000000001));
#107519=CARTESIAN_POINT('Origin',(-0.0203762178069016,0.00227581852804817,
0.05660000000001));
#107520=CARTESIAN_POINT('Origin',(-0.0203762178068916,0.00227581852803817,
0.0566));
#107521=CARTESIAN_POINT('',(-0.0135678120097901,-0.00938160873967384,0.06075));
#107522=CARTESIAN_POINT('',(-0.0135678120098001,-0.00938160873968384,0.06075000000001));
#107523=CARTESIAN_POINT('Origin',(-0.0203762178069016,0.00227581852804817,
0.06075000000001));
#107524=CARTESIAN_POINT('Origin',(-0.0203762178069016,0.00227581852804817,
0.05525000000001));
#107525=CARTESIAN_POINT('Origin',(-0.0031262178068916,0.00227581852803817,
0.0586));
#107526=CARTESIAN_POINT('',(-0.00647621780689159,0.0158691073133175,0.0586));
#107527=CARTESIAN_POINT('Origin',(-0.00312621780690161,0.00227581852804816,
0.05860000000001));
#107528=CARTESIAN_POINT('',(-0.00647621780690159,0.0158691073133275,0.05860000000001));
#107529=CARTESIAN_POINT('Origin',(-0.0339352129125134,-0.0163741814719618,
0.0566));
#107530=CARTESIAN_POINT('',(0.00785982116242948,-0.0163741814719618,0.06075));
#107531=CARTESIAN_POINT('',(0.00785982116243948,-0.0163741814719718,0.06075000000001));
#107532=CARTESIAN_POINT('',(0.00785982116242948,-0.0163741814719618,0.05525));
#107533=CARTESIAN_POINT('',(0.00785982116243948,-0.0163741814719718,0.05660000000001));
#107534=CARTESIAN_POINT('',(-0.0339352129125234,-0.0163741814719718,0.05525000000001));
#107535=CARTESIAN_POINT('Origin',(-0.0339352129125134,-0.0163741814719618,
0.0566));
#107536=CARTESIAN_POINT('',(-0.0194688327842092,-0.0163741814719618,0.05525));
#107537=CARTESIAN_POINT('',(-0.0339352129125134,-0.0163741814719618,0.05525));
#107538=CARTESIAN_POINT('',(-0.0339352129125234,-0.0163741814719718,0.05525000000001));
#107539=CARTESIAN_POINT('',(-0.0339352129125134,-0.0163741814719618,0.0655));
#107540=CARTESIAN_POINT('',(-0.0339352129125234,-0.0163741814719718,0.05660000000001));
#107541=CARTESIAN_POINT('',(-0.0330326892153179,-0.0163741814719618,0.0655));
#107542=CARTESIAN_POINT('',(-0.0330326892153278,-0.0163741814719718,0.06550000000001));
#107543=CARTESIAN_POINT('',(-0.0330326892153179,-0.0163741814719618,0.0615));
#107544=CARTESIAN_POINT('',(-0.0330326892153278,-0.0163741814719718,0.06550000000001));
#107545=CARTESIAN_POINT('',(-0.0194688327842092,-0.0163741814719618,0.0615));
#107546=CARTESIAN_POINT('',(-0.0330326892153278,-0.0163741814719718,0.06150000000001));
#107547=CARTESIAN_POINT('',(-0.0194688327842192,-0.0163741814719718,0.0450676623509237));
#107548=CARTESIAN_POINT('Origin',(-0.0411262178068916,-0.0184741814719619,
0.08925));
#107549=CARTESIAN_POINT('',(0.0108737821931084,-0.0145623019693,0.08925));
#107550=CARTESIAN_POINT('',(0.0108737821931084,0.00675805157507176,0.08925));
#107551=CARTESIAN_POINT('',(0.0108737821931184,-0.0184741814719718,0.08925000000001));
#107552=CARTESIAN_POINT('',(-0.00414398475985796,0.0217758185280382,0.08925));
#107553=CARTESIAN_POINT('',(-0.00251010128338471,0.0201419350515649,0.08925000000001));
#107554=CARTESIAN_POINT('',(-0.0372143383042298,0.0217758185280382,0.08925));
#107555=CARTESIAN_POINT('',(-0.0411262178069016,0.0217758185280482,0.08925000000001));
#107556=CARTESIAN_POINT('',(-0.0398762178068916,0.0191139390253764,0.08925));
#107557=CARTESIAN_POINT('',(-0.0592952780555707,-0.00030512122330272,0.08925000000001));
#107558=CARTESIAN_POINT('',(-0.0398762178068916,-0.0145623019693,0.08925));
#107559=CARTESIAN_POINT('',(-0.0398762178069016,-0.0184741814719718,0.08925000000001));
#107560=CARTESIAN_POINT('',(-0.0372143383042298,-0.0172241814719618,0.08925));
#107561=CARTESIAN_POINT('',(-0.0385452780555707,-0.0158932417206409,0.08925000000001));
#107562=CARTESIAN_POINT('',(0.00821190269044663,-0.0172241814719618,0.08925));
#107563=CARTESIAN_POINT('',(-0.0411262178069016,-0.0172241814719718,0.08925000000001));
#107564=CARTESIAN_POINT('',(-0.0170821575582324,-0.0425182417206409,0.08925000000001));
#107565=CARTESIAN_POINT('',(-0.0266262178068916,0.0142758185280382,0.08925));
#107566=CARTESIAN_POINT('',(-0.0266262178068916,-0.00972418147196183,0.08925));
#107567=CARTESIAN_POINT('',(-0.0266262178069016,-0.00972418147197183,0.08925000000001));
#107568=CARTESIAN_POINT('',(-0.0246762178068916,0.0202758185280381,0.08925));
#107569=CARTESIAN_POINT('',(-0.0266262178069016,0.0142758185280482,0.08925000000001));
#107570=CARTESIAN_POINT('',(-0.0166762178068916,0.0202758185280381,0.08925));
#107571=CARTESIAN_POINT('',(-0.0246762178069016,0.0202758185280481,0.08925000000001));
#107572=CARTESIAN_POINT('',(-0.0147262178068916,0.0142758185280382,0.08925));
#107573=CARTESIAN_POINT('',(-0.0166762178069016,0.0202758185280481,0.08925000000001));
#107574=CARTESIAN_POINT('',(-0.0147262178068916,-0.00972418147196183,0.08925));
#107575=CARTESIAN_POINT('',(-0.0147262178069016,0.0142758185280482,0.08925000000001));
#107576=CARTESIAN_POINT('',(-0.0166762178068916,-0.0157241814719619,0.08925));
#107577=CARTESIAN_POINT('',(-0.0147262178069016,-0.00972418147197183,0.08925000000001));
#107578=CARTESIAN_POINT('',(-0.0246762178068916,-0.0157241814719619,0.08925));
#107579=CARTESIAN_POINT('',(-0.0166762178069016,-0.0157241814719719,0.08925000000001));
#107580=CARTESIAN_POINT('',(-0.0246762178069016,-0.0157241814719719,0.08925000000001));
#107581=CARTESIAN_POINT('Origin',(-0.0411262178068916,-0.0184741814719619,
0.05525));
#107582=CARTESIAN_POINT('',(0.00872966964341299,-0.0155043329909783,0.05525));
#107583=CARTESIAN_POINT('',(0.00785982116243948,-0.0163741814719718,0.05525000000001));
#107584=CARTESIAN_POINT('',(0.00872966964341299,-0.0184741814719618,0.05525));
#107585=CARTESIAN_POINT('',(0.00872966964342298,0.0230258185280482,0.05525000000001));
#107586=CARTESIAN_POINT('',(-0.0377321052571961,-0.0184741814719619,0.05525));
#107587=CARTESIAN_POINT('',(0.00872966964342298,-0.0184741814719718,0.05525000000001));
#107588=CARTESIAN_POINT('',(-0.0411262178068916,-0.0150800689222664,0.05525));
#107589=CARTESIAN_POINT('',(-0.0377321052572061,-0.0184741814719718,0.05525000000001));
#107590=CARTESIAN_POINT('',(-0.0411262178068916,0.0196317059783427,0.05525));
#107591=CARTESIAN_POINT('',(-0.0411262178069016,-0.0150800689222764,0.05525000000001));
#107592=CARTESIAN_POINT('',(-0.0377321052571961,0.0230258185280382,0.05525));
#107593=CARTESIAN_POINT('',(-0.0411262178069016,0.0196317059783527,0.05525000000001));
#107594=CARTESIAN_POINT('',(-0.00362621780689159,0.0230258185280382,0.05525));
#107595=CARTESIAN_POINT('',(-0.0377321052572061,0.0230258185280482,0.05525000000001));
#107596=CARTESIAN_POINT('',(0.000873782193108408,0.0185258185280382,0.05525));
#107597=CARTESIAN_POINT('',(-0.0036262178069016,0.0230258185280482,0.05525000000001));
#107598=CARTESIAN_POINT('',(0.000873782193108401,0.0102484278875892,0.05525));
#107599=CARTESIAN_POINT('',(0.000873782193118408,0.0185258185280481,0.05525000000001));
#107600=CARTESIAN_POINT('',(0.00180163765660117,0.00768680185188279,0.05525));
#107601=CARTESIAN_POINT('Origin',(0.0048737821931184,0.0102484278875992,
0.05525000000001));
#107602=CARTESIAN_POINT('',(0.00244204416552777,0.00691876571775598,0.05525));
#107603=CARTESIAN_POINT('',(0.00244204416553777,0.00691876571776598,0.05525000000001));
#107604=CARTESIAN_POINT('',(0.0041237821931084,0.00227581852803816,0.05525));
#107605=CARTESIAN_POINT('Origin',(-0.00312621780690161,0.00227581852804816,
0.05525000000001));
#107606=CARTESIAN_POINT('',(0.0041237821931084,-0.00233742823514713,0.05525));
#107607=CARTESIAN_POINT('',(0.00412378219311839,0.00227581852804816,0.05525000000001));
#107608=CARTESIAN_POINT('',(0.00500246184954876,-0.00445874857870678,0.05525));
#107609=CARTESIAN_POINT('Origin',(0.00712378219311841,-0.00233742823515713,
0.05525000000001));
#107610=CARTESIAN_POINT('',(0.00872966964341298,-0.00818595637257098,0.05525));
#107611=CARTESIAN_POINT('',(0.00500246184955876,-0.00445874857871678,0.05525000000001));
#107612=CARTESIAN_POINT('',(0.00872966964341299,-0.0110143834973172,0.05525));
#107613=CARTESIAN_POINT('',(0.00872966964342298,0.0230258185280482,0.05525000000001));
#107614=CARTESIAN_POINT('',(0.00358824828717567,-0.00587296214107986,0.05525));
#107615=CARTESIAN_POINT('',(0.0100237821931184,-0.0123084960470226,0.05525000000001));
#107616=CARTESIAN_POINT('',(0.0021237821931084,-0.00233742823514713,0.05525));
#107617=CARTESIAN_POINT('Origin',(0.00712378219311841,-0.00233742823515713,
0.05525000000001));
#107618=CARTESIAN_POINT('',(0.0021237821931084,0.00227581852803816,0.05525));
#107619=CARTESIAN_POINT('',(0.0021237821931184,0.00227581852804816,0.05525000000001));
#107620=CARTESIAN_POINT('',(0.000905971897274149,0.00563795269990278,0.05525));
#107621=CARTESIAN_POINT('Origin',(-0.0031262178069016,0.00227581852804816,
0.05525000000001));
#107622=CARTESIAN_POINT('',(0.000282704463412254,0.00638543403208472,0.05525));
#107623=CARTESIAN_POINT('',(0.000905971897284156,0.00563795269991278,0.05525000000001));
#107624=CARTESIAN_POINT('',(-0.0012262178068916,0.0105512709814273,0.05525));
#107625=CARTESIAN_POINT('Origin',(0.00527877065166022,0.0105512709814373,
0.05525000000001));
#107626=CARTESIAN_POINT('',(-0.0012262178069016,0.0105512709814373,0.05525000000001));
#107627=CARTESIAN_POINT('',(-0.0339352129125134,0.0209258185280382,0.05525));
#107628=CARTESIAN_POINT('',(-0.00681722270127977,0.0209258185280481,0.05525000000001));
#107629=CARTESIAN_POINT('',(-0.0390262178068916,0.01583481363366,0.05525));
#107630=CARTESIAN_POINT('Origin',(-0.0358762178069016,0.0177758185280482,
0.05525000000001));
#107631=CARTESIAN_POINT('',(-0.0390262178068916,-0.0112831765775837,0.05525));
#107632=CARTESIAN_POINT('',(-0.0390262178069016,0.01583481363367,0.05525000000001));
#107633=CARTESIAN_POINT('Origin',(-0.0358762178069016,-0.0132241814719718,
0.05525000000001));
#107634=CARTESIAN_POINT('Origin',(-0.0186262178069016,-0.0128741814719718,
0.05525000000001));
#107635=CARTESIAN_POINT('Origin',(-0.0377321052571961,-0.0184741814719619,
0.08925));
#107636=CARTESIAN_POINT('',(-0.0377321052571961,-0.0184741814719619,0.088));
#107637=CARTESIAN_POINT('',(-0.0377321052572061,-0.0184741814719718,0.08925000000001));
#107638=CARTESIAN_POINT('',(-0.0411262178068916,-0.0150800689222664,0.088));
#107639=CARTESIAN_POINT('',(-0.0377321052572061,-0.0184741814719718,0.08800000000001));
#107640=CARTESIAN_POINT('',(-0.0411262178069016,-0.0150800689222764,0.08925000000001));
#107641=CARTESIAN_POINT('Origin',(0.00872966964341299,-0.0184741814719619,
0.08925));
#107642=CARTESIAN_POINT('',(0.0121237821931184,-0.0184741814719718,0.0829760869565317));
#107643=CARTESIAN_POINT('',(0.00872966964342298,-0.0184741814719718,0.08800000000001));
#107644=CARTESIAN_POINT('',(0.00872966964341299,-0.0184741814719618,0.0647218269911845));
#107645=CARTESIAN_POINT('',(0.00872966964342298,-0.0184741814719718,0.08925000000001));
#107646=CARTESIAN_POINT('',(0.0021237821931184,-0.0184741814719718,0.06355000000001));
#107647=CARTESIAN_POINT('',(-0.0311262178069016,-0.0184741814719718,0.06355000000001));
#107648=CARTESIAN_POINT('Origin',(0.0121237821931084,-0.0150800689222664,
0.08925));
#107649=CARTESIAN_POINT('',(0.0121237821931084,-0.0150800689222664,0.0653239130434783));
#107650=CARTESIAN_POINT('',(0.0121237821931084,-0.0150800689222664,0.0586441125496955));
#107651=CARTESIAN_POINT('',(0.0121237821931184,-0.0150800689222764,0.08925000000001));
#107652=CARTESIAN_POINT('',(0.0142130498815413,-0.0129908012338535,0.0656945309638694));
#107653=CARTESIAN_POINT('',(0.0223257446765532,-0.0048781064388415,0.0688460750331404));
#107654=CARTESIAN_POINT('Origin',(0.0121237821931084,0.00427931609139309,
0.08925));
#107655=CARTESIAN_POINT('',(0.0121237821931184,-0.0144741814719718,0.0829760869565317));
#107656=CARTESIAN_POINT('',(0.0121237821931184,-0.0144741814719718,0.0653239130434883));
#107657=CARTESIAN_POINT('',(0.0121237821931084,-0.0115800689222664,0.0586441125496955));
#107658=CARTESIAN_POINT('',(0.0121237821931184,0.0230258185280482,0.0586441125497055));
#107659=CARTESIAN_POINT('',(0.0121237821931184,-0.0115800689222764,0.0998391810594335));
#107660=CARTESIAN_POINT('',(0.0121237821931084,0.00427931609139309,0.088));
#107661=CARTESIAN_POINT('',(0.0121237821931184,0.00427931609140309,0.08925000000001));
#107662=CARTESIAN_POINT('',(0.0121237821931184,0.00427931609140309,0.08800000000001));
#107663=CARTESIAN_POINT('Origin',(0.0112230245980259,0.00817657612312065,
0.08925));
#107664=CARTESIAN_POINT('',(0.0112230245980259,0.00817657612312065,0.088));
#107665=CARTESIAN_POINT('',(0.0112230245980359,0.00817657612313065,0.08925000000001));
#107666=CARTESIAN_POINT('',(0.0114917234185988,0.00701401121141935,0.0886320587745096));
#107667=CARTESIAN_POINT('',(0.00874560658929598,0.018895489002749,0.0821723830896977));
#107668=CARTESIAN_POINT('',(0.0167544258428938,-0.0157558437740066,0.0833693563502346));
#107669=CARTESIAN_POINT('Origin',(-0.00362621780689159,0.0230258185280382,
0.08925));
#107670=CARTESIAN_POINT('',(0.000873782193118408,0.0185258185280481,0.0998391810594335));
#107671=CARTESIAN_POINT('',(-0.00362621780689159,0.0230258185280382,0.088));
#107672=CARTESIAN_POINT('',(-0.0036262178069016,0.0230258185280482,0.08925000000001));
#107673=CARTESIAN_POINT('',(-0.0036262178069016,0.0230258185280482,0.08800000000001));
#107674=CARTESIAN_POINT('Origin',(-0.0377321052571961,0.0230258185280382,
0.08925));
#107675=CARTESIAN_POINT('',(-0.0377321052571961,0.0230258185280382,0.088));
#107676=CARTESIAN_POINT('',(-0.0377321052572061,0.0230258185280482,0.08925000000001));
#107677=CARTESIAN_POINT('',(-0.0377321052572061,0.0230258185280482,0.08800000000001));
#107678=CARTESIAN_POINT('Origin',(-0.0411262178068916,0.0196317059783427,
0.08925));
#107679=CARTESIAN_POINT('',(-0.0411262178068916,0.0196317059783427,0.088));
#107680=CARTESIAN_POINT('',(-0.0411262178069016,0.0196317059783527,0.08925000000001));
#107681=CARTESIAN_POINT('',(-0.0411262178069016,0.0196317059783527,0.08800000000001));
#107682=CARTESIAN_POINT('Origin',(-0.0411262178068916,-0.0150800689222664,
0.08925));
#107683=CARTESIAN_POINT('',(-0.0411262178069016,-0.0150800689222764,0.08800000000001));
#107684=CARTESIAN_POINT('Origin',(-0.0385452780555607,-0.0158932417206309,
0.08925));
#107685=CARTESIAN_POINT('',(-0.0406223836679862,-0.0148713739887511,0.0885038341389253));
#107686=CARTESIAN_POINT('',(-0.0370656257560876,-0.0168651576213277,0.0896090238506542));
#107687=CARTESIAN_POINT('Origin',(-0.0411262178068916,-0.0172241814719618,
0.08925));
#107688=CARTESIAN_POINT('',(0.00431376816786663,-0.00781325223958014,0.0986609292324018));
#107689=CARTESIAN_POINT('Origin',(-0.0398762178068916,-0.0184741814719619,
0.08925));
#107690=CARTESIAN_POINT('',(-0.045114550931596,0.0212837276498631,0.0840116668753155));
#107691=CARTESIAN_POINT('Origin',(-0.0170821575582224,-0.0425182417206309,
0.08925));
#107692=CARTESIAN_POINT('',(0.00333260752472027,-0.0114386451454352,0.0967911746684082));
#107693=CARTESIAN_POINT('Origin',(-0.0592952780555607,-0.00030512122329272,
0.08925));
#107694=CARTESIAN_POINT('',(-0.0375234103236808,0.0225219843891328,0.0885038341389253));
#107695=CARTESIAN_POINT('Origin',(0.0108737821931084,-0.0184741814719619,
0.08925));
#107696=CARTESIAN_POINT('',(0.00726345093845756,0.00526260340474177,0.0928603312546709));
#107697=CARTESIAN_POINT('Origin',(-0.0411262178068916,0.0217758185280382,
0.08925));
#107698=CARTESIAN_POINT('',(-0.00706589823995062,0.0147216953763519,0.0963041231517064));
#107699=CARTESIAN_POINT('Origin',(-0.00251010128337472,0.020141935051555,
0.08925));
#107700=CARTESIAN_POINT('Origin',(-0.0358762178068916,-0.0132241814719618,
0.08545));
#107701=CARTESIAN_POINT('Origin',(-0.00487621780689159,0.0177758185280382,
0.08545));
#107702=CARTESIAN_POINT('Origin',(-0.0358762178068916,0.0177758185280382,
0.08545));
#107703=CARTESIAN_POINT('Origin',(0.00500246184954876,-0.00445874857870678,
0.0998391810594235));
#107704=CARTESIAN_POINT('',(0.0211079248006548,-0.0205642115298128,0.0676282551572419));
#107705=CARTESIAN_POINT('',(0.00500246184954876,-0.00445874857870678,0.0586));
#107706=CARTESIAN_POINT('',(0.00500246184955876,-0.00445874857871678,0.0998391810594335));
#107707=CARTESIAN_POINT('',(0.00500246184955876,-0.00445874857871678,0.05860000000001));
#107708=CARTESIAN_POINT('Origin',(0.00712378219310841,-0.00233742823514713,
0.0998391810594235));
#107709=CARTESIAN_POINT('',(0.0041237821931084,-0.00233742823514714,0.0586));
#107710=CARTESIAN_POINT('',(0.0041237821931184,-0.00233742823515713,0.0998391810594335));
#107711=CARTESIAN_POINT('Origin',(0.00712378219311841,-0.00233742823515713,
0.05860000000001));
#107712=CARTESIAN_POINT('Origin',(0.00412378219310839,0.00227581852803816,
0.0998391810594235));
#107713=CARTESIAN_POINT('',(0.0041237821931084,0.00227581852803816,0.0586));
#107714=CARTESIAN_POINT('',(0.0041237821931184,0.00227581852804816,0.0998391810594335));
#107715=CARTESIAN_POINT('',(0.00412378219311839,0.00227581852804816,0.05860000000001));
#107716=CARTESIAN_POINT('Origin',(-0.0031262178068916,0.00227581852803817,
0.0998391810594235));
#107717=CARTESIAN_POINT('',(0.00244204416552777,0.00691876571775598,0.0586));
#107718=CARTESIAN_POINT('',(0.00244204416553777,0.00691876571776598,0.0998391810594335));
#107719=CARTESIAN_POINT('Origin',(-0.00312621780690161,0.00227581852804816,
0.05860000000001));
#107720=CARTESIAN_POINT('Origin',(0.00244204416552777,0.00691876571775598,
0.0998391810594235));
#107721=CARTESIAN_POINT('',(0.00180163765660117,0.00768680185188279,0.0586));
#107722=CARTESIAN_POINT('',(0.00180163765661117,0.00768680185189279,0.0998391810594335));
#107723=CARTESIAN_POINT('',(0.00244204416553777,0.00691876571776598,0.05860000000001));
#107724=CARTESIAN_POINT('Origin',(0.0048737821931084,0.0102484278875892,
0.0998391810594235));
#107725=CARTESIAN_POINT('',(0.000873782193108401,0.0102484278875892,0.0586));
#107726=CARTESIAN_POINT('',(0.000873782193118401,0.0102484278875992,0.0998391810594335));
#107727=CARTESIAN_POINT('Origin',(0.0048737821931184,0.0102484278875992,
0.05860000000001));
#107728=CARTESIAN_POINT('Origin',(0.000873782193108408,0.0185258185280382,
0.0998391810594235));
#107729=CARTESIAN_POINT('',(0.000873782193108408,0.0156922263930369,0.0586));
#107730=CARTESIAN_POINT('',(0.000873782193118408,0.0156922263930469,0.05860000000001));
#107731=CARTESIAN_POINT('',(0.000873782193118408,0.0185258185280481,0.05860000000001));
#107732=CARTESIAN_POINT('Origin',(-0.0031262178068916,0.00227581852803817,
0.0586));
#107733=CARTESIAN_POINT('',(-0.00327621780689159,0.0162750149335466,0.0586));
#107734=CARTESIAN_POINT('',(-0.0032762178069016,0.0162750149335566,0.05860000000001));
#107735=CARTESIAN_POINT('Origin',(-0.00312621780690161,0.00227581852804816,
0.05860000000001));
#107736=CARTESIAN_POINT('Origin',(-0.0031262178068916,0.00227581852803817,
0.0586));
#107737=CARTESIAN_POINT('',(-0.0032762178069016,0.0177758185280482,0.05860000000001));
#107738=CARTESIAN_POINT('',(-0.00647621780690159,0.0177758185280482,0.05860000000001));
#107739=CARTESIAN_POINT('Origin',(-0.00327621780689159,0.0177758185280382,
0.0586));
#107740=CARTESIAN_POINT('Origin',(-0.00647621780689159,0.0177758185280382,
0.0586));
#107741=CARTESIAN_POINT('Origin',(-0.00681722270126977,0.0209258185280382,
0.0566));
#107742=CARTESIAN_POINT('',(-0.0339352129125134,0.0209258185280382,0.0655));
#107743=CARTESIAN_POINT('',(-0.00681722270127977,0.0209258185280481,0.06550000000001));
#107744=CARTESIAN_POINT('',(-0.0339352129125234,0.0209258185280481,0.05660000000001));
#107745=CARTESIAN_POINT('Origin',(-0.0358762178068916,0.0177758185280382,
0.0566));
#107746=CARTESIAN_POINT('',(-0.0390262178068916,0.01583481363366,0.0655));
#107747=CARTESIAN_POINT('Origin',(-0.0358762178069016,0.0177758185280482,
0.06550000000001));
#107748=CARTESIAN_POINT('',(-0.0390262178069016,0.01583481363367,0.05660000000001));
#107749=CARTESIAN_POINT('Origin',(-0.0390262178068916,0.01583481363366,
0.0566));
#107750=CARTESIAN_POINT('',(-0.0390262178068916,-0.0112831765775837,0.0655));
#107751=CARTESIAN_POINT('',(-0.0390262178069016,0.01583481363367,0.06550000000001));
#107752=CARTESIAN_POINT('',(-0.0390262178069016,-0.0112831765775937,0.05660000000001));
#107753=CARTESIAN_POINT('Origin',(-0.0358762178068916,-0.0132241814719618,
0.0566));
#107754=CARTESIAN_POINT('Origin',(-0.0358762178069016,-0.0132241814719718,
0.06550000000001));
#107755=CARTESIAN_POINT('Origin',(0.00785982116242948,-0.0163741814719618,
0.0566));
#107756=CARTESIAN_POINT('',(0.0100237821931084,-0.0142102204412829,0.06075));
#107757=CARTESIAN_POINT('',(0.0100237821931084,-0.0142102204412829,0.0565441125496954));
#107758=CARTESIAN_POINT('',(0.0100237821931184,-0.0142102204412929,0.05660000000001));
#107759=CARTESIAN_POINT('',(0.00859977065610065,-0.0156342319783106,0.0551201010126877));
#107760=CARTESIAN_POINT('',(0.0100237821931184,-0.0142102204412929,0.06075000000001));
#107761=CARTESIAN_POINT('Origin',(0.0100237821931084,-0.0142102204412829,
0.0566));
#107762=CARTESIAN_POINT('',(0.0100237821931084,-0.0123084960470126,0.06075));
#107763=CARTESIAN_POINT('',(0.0100237821931084,-0.0123084960470126,0.0565441125496954));
#107764=CARTESIAN_POINT('',(0.0100237821931184,-0.0123084960470226,0.05660000000001));
#107765=CARTESIAN_POINT('',(0.0100237821931184,-0.0142102204412929,0.0565441125497054));
#107766=CARTESIAN_POINT('',(0.0100237821931184,-0.0123084960470226,0.06075000000001));
#107767=CARTESIAN_POINT('Origin',(0.0100237821931084,-0.0123084960470126,
0.0566));
#107768=CARTESIAN_POINT('',(0.0100424113432199,-0.0123271251971241,0.056562741699807));
#107769=CARTESIAN_POINT('',(0.00719958354106424,-0.00948429739496843,0.06075));
#107770=CARTESIAN_POINT('',(0.00719958354107424,-0.00948429739497843,0.06075000000001));
#107771=CARTESIAN_POINT('',(0.00719958354107424,-0.00948429739497843,0.06075000000001));
#107772=CARTESIAN_POINT('',(0.00358824828718567,-0.00587296214108986,0.05660000000001));
#107773=CARTESIAN_POINT('Origin',(0.00712378219310841,-0.00233742823514713,
0.0566));
#107774=CARTESIAN_POINT('',(0.0021237821931184,-0.00233742823515713,0.05660000000001));
#107775=CARTESIAN_POINT('Origin',(0.0021237821931084,0.00227581852803816,
0.0566));
#107776=CARTESIAN_POINT('',(0.0021237821931184,0.00227581852804816,0.05660000000001));
#107777=CARTESIAN_POINT('Origin',(-0.00312621780689159,0.00227581852803816,
0.0566));
#107778=CARTESIAN_POINT('',(0.000905971897284149,0.00563795269991278,0.05660000000001));
#107779=CARTESIAN_POINT('Origin',(0.000905971897274156,0.00563795269990278,
0.0566));
#107780=CARTESIAN_POINT('',(0.000282704463422255,0.00638543403209472,0.05660000000001));
#107781=CARTESIAN_POINT('Origin',(0.00527877065165022,0.0105512709814273,
0.0566));
#107782=CARTESIAN_POINT('',(-0.0012262178069016,0.0105512709814373,0.05660000000001));
#107783=CARTESIAN_POINT('Origin',(-0.0012262178068916,0.0105512709814273,
0.0566));
#107784=CARTESIAN_POINT('Origin',(0.0121237821931084,0.0230258185280382,
0.0586441125496955));
#107785=CARTESIAN_POINT('Origin',(-0.0186262178068916,-0.0128741814719618,
0.0450676623509137));
#107786=CARTESIAN_POINT('Origin',(-0.0186262178069016,-0.0128741814719718,
0.06150000000001));
#107787=CARTESIAN_POINT('Origin',(-0.00487621780689159,0.0177758185280382,
0.0566));
#107788=CARTESIAN_POINT('Origin',(-0.0203762178068916,0.00227581852803817,
0.0615));
#107789=CARTESIAN_POINT('',(-0.0256278910010042,-0.0101608180213908,0.06150000000001));
#107790=CARTESIAN_POINT('Origin',(-0.0203762178068916,0.00227581852803817,
0.0737));
#107791=CARTESIAN_POINT('Origin',(-0.0203762178068916,0.00227581852803817,
0.0862));
#107792=CARTESIAN_POINT('Origin',(-0.00487621780689159,0.0177758185280382,
0.0566));
#107793=CARTESIAN_POINT('Origin',(-0.0266262178068916,0.0142758185280382,
0.08775));
#107794=CARTESIAN_POINT('',(-0.0266262178068916,0.0142758185280382,0.08775));
#107795=CARTESIAN_POINT('',(-0.0266262178069016,0.0142758185280482,0.08775000000001));
#107796=CARTESIAN_POINT('',(-0.0246762178068916,0.0202758185280381,0.08775));
#107797=CARTESIAN_POINT('',(-0.0266262178069016,0.0142758185280482,0.08775000000001));
#107798=CARTESIAN_POINT('',(-0.0246762178069016,0.0202758185280481,0.08775000000001));
#107799=CARTESIAN_POINT('Origin',(-0.0246762178068916,0.0202758185280381,
0.08775));
#107800=CARTESIAN_POINT('',(-0.0166762178068916,0.0202758185280381,0.08775));
#107801=CARTESIAN_POINT('',(-0.0246762178069016,0.0202758185280481,0.08775000000001));
#107802=CARTESIAN_POINT('',(-0.0166762178069016,0.0202758185280481,0.08775000000001));
#107803=CARTESIAN_POINT('Origin',(-0.0166762178068916,0.0202758185280381,
0.08775));
#107804=CARTESIAN_POINT('',(-0.0147262178068916,0.0142758185280382,0.08775));
#107805=CARTESIAN_POINT('',(-0.0166762178069016,0.0202758185280481,0.08775000000001));
#107806=CARTESIAN_POINT('',(-0.0147262178069016,0.0142758185280482,0.08775000000001));
#107807=CARTESIAN_POINT('Origin',(-0.0147262178068916,0.0142758185280382,
0.08775));
#107808=CARTESIAN_POINT('',(-0.0147262178068916,-0.00972418147196183,0.08775));
#107809=CARTESIAN_POINT('',(-0.0147262178069016,0.0142758185280482,0.08775000000001));
#107810=CARTESIAN_POINT('',(-0.0147262178069016,-0.00972418147197183,0.08775000000001));
#107811=CARTESIAN_POINT('Origin',(-0.0147262178068916,-0.00972418147196183,
0.08775));
#107812=CARTESIAN_POINT('',(-0.0166762178068916,-0.0157241814719619,0.08775));
#107813=CARTESIAN_POINT('',(-0.0147262178069016,-0.00972418147197183,0.08775000000001));
#107814=CARTESIAN_POINT('',(-0.0166762178069016,-0.0157241814719719,0.08775000000001));
#107815=CARTESIAN_POINT('Origin',(-0.0166762178068916,-0.0157241814719619,
0.08775));
#107816=CARTESIAN_POINT('',(-0.0246762178068916,-0.0157241814719619,0.08775));
#107817=CARTESIAN_POINT('',(-0.0166762178069016,-0.0157241814719719,0.08775000000001));
#107818=CARTESIAN_POINT('',(-0.0246762178069016,-0.0157241814719719,0.08775000000001));
#107819=CARTESIAN_POINT('Origin',(-0.0246762178068916,-0.0157241814719619,
0.08775));
#107820=CARTESIAN_POINT('',(-0.0266262178068916,-0.00972418147196183,0.08775));
#107821=CARTESIAN_POINT('',(-0.0246762178069016,-0.0157241814719719,0.08775000000001));
#107822=CARTESIAN_POINT('',(-0.0266262178069016,-0.00972418147197183,0.08775000000001));
#107823=CARTESIAN_POINT('Origin',(-0.0266262178068916,-0.00972418147196183,
0.08775));
#107824=CARTESIAN_POINT('',(-0.0266262178069016,-0.00972418147197183,0.08775000000001));
#107825=CARTESIAN_POINT('Origin',(-0.0411262178068916,-0.0184741814719619,
0.08775));
#107826=CARTESIAN_POINT('Origin',(-0.00312621780689159,0.00227581852803817,
0.06075));
#107827=CARTESIAN_POINT('Origin',(-0.0031262178069016,0.00227581852804816,
0.06075000000001));
#107828=CARTESIAN_POINT('Origin',(-0.00312621780689159,0.00227581852803817,
0.06075));
#107829=CARTESIAN_POINT('Origin',(-0.0256278910009942,-0.0101608180213808,
0.0655));
#107830=CARTESIAN_POINT('',(-0.0311262178068916,-0.0147744620163014,0.0655));
#107831=CARTESIAN_POINT('',(-0.0256278910010042,-0.0101608180213908,0.06550000000001));
#107832=CARTESIAN_POINT('',(-0.0311262178068916,-0.0147744620163014,0.06355));
#107833=CARTESIAN_POINT('',(-0.0311262178069016,-0.0147744620163114,0.06550000000001));
#107834=CARTESIAN_POINT('',(-0.0307683573893888,-0.0144741814719618,0.06355));
#107835=CARTESIAN_POINT('',(-0.0256278910010042,-0.0101608180213908,0.06355000000001));
#107836=CARTESIAN_POINT('',(-0.0307683573893888,-0.0144741814719618,0.0655));
#107837=CARTESIAN_POINT('',(-0.0307683573893988,-0.0144741814719718,0.06550000000001));
#107838=CARTESIAN_POINT('',(-0.0256278910010042,-0.0101608180213908,0.06550000000001));
#107839=CARTESIAN_POINT('Origin',(-0.00312621780689159,0.00227581852803817,
0.0655));
#107840=CARTESIAN_POINT('Origin',(-0.0031262178069016,0.00227581852804816,
0.06550000000001));
#107841=CARTESIAN_POINT('Origin',(-0.00487621780689159,0.0177758185280382,
0.0655));
#107842=CARTESIAN_POINT('',(-0.0311262178068916,-0.0144741814719618,0.0655));
#107843=CARTESIAN_POINT('',(-0.0311262178069016,0.0177758185280482,0.06550000000001));
#107844=CARTESIAN_POINT('',(-0.00487621780690158,-0.0144741814719718,0.06550000000001));
#107845=CARTESIAN_POINT('Origin',(0.0121237821931084,-0.0144741814719618,
0.0829760869565217));
#107846=CARTESIAN_POINT('Origin',(0.0021237821931084,-0.0144741814719618,
0.06355));
#107847=CARTESIAN_POINT('Origin',(-0.0311262178068916,-0.0184741814719619,
0.0578931457505076));
#107848=CARTESIAN_POINT('',(-0.0171262178069015,-0.00447418147197182,0.0326378260227564));
#107849=CARTESIAN_POINT('Origin',(-0.0311262178068916,-0.0144741814719618,
0.06355));
#107850=CARTESIAN_POINT('',(-0.0311262178068916,-0.0144741814719618,0.06355));
#107851=CARTESIAN_POINT('',(-0.0311262178069016,-0.0144741814719718,0.06355000000001));
#107852=CARTESIAN_POINT('',(-0.0271262178069016,-0.0144741814719718,0.06355000000001));
#107853=CARTESIAN_POINT('Origin',(-0.0311262178068916,-0.0144741814719618,
0.0578931457505076));
#107854=CARTESIAN_POINT('',(-0.0311262178069016,-0.0144741814719718,0.0578931457505176));
#107855=CARTESIAN_POINT('Origin',(-0.0271262178068916,-0.0144741814719618,
0.0578931457505076));
#107856=CARTESIAN_POINT('Origin',(-0.0171262178068915,-0.00447418147196182,
0.0326378260227464));
#107857=CARTESIAN_POINT('',(0.0021237821931184,-0.00447418147197182,0.0326378260227564));
#107858=CARTESIAN_POINT('Origin',(0.0021237821931084,-0.00447418147196182,
0.0326378260227464));
#107859=CARTESIAN_POINT('Origin',(-0.0286262178068916,-0.00152418147196182,
0.071));
#107860=CARTESIAN_POINT('Origin',(-0.0381262178068916,-0.00152418147196182,
0.071));
#107861=CARTESIAN_POINT('',(-0.0381262178068916,0.00247581852803818,0.0834721359549996));
#107862=CARTESIAN_POINT('',(-0.0381262178068916,-0.00552418147196183,0.0834721359549996));
#107863=CARTESIAN_POINT('Origin',(-0.0381262178069016,-0.00152418147197183,
0.07900000000001));
#107864=CARTESIAN_POINT('',(-0.0381262178069016,0.00247581852804817,0.0819282032302855));
#107865=CARTESIAN_POINT('',(-0.0381262178069016,-0.00552418147197183,0.0859282032302855));
#107866=CARTESIAN_POINT('Origin',(-0.0411262178068916,-0.00152418147196182,
0.079));
#107867=CARTESIAN_POINT('',(-0.0321262178068916,0.00247581852803818,0.0834721359549996));
#107868=CARTESIAN_POINT('',(-0.0321262178068916,-0.00552418147196183,0.0834721359549996));
#107869=CARTESIAN_POINT('Origin',(-0.0321262178069016,-0.00152418147197183,
0.07900000000001));
#107870=CARTESIAN_POINT('',(-0.0411262178069016,0.00247581852804817,0.0834721359550096));
#107871=CARTESIAN_POINT('',(-0.0411262178069016,-0.00552418147197183,0.0834721359550096));
#107872=CARTESIAN_POINT('Origin',(-0.0321262178068916,-0.00152418147196182,
0.073));
#107873=CARTESIAN_POINT('',(-0.0321262178069016,0.00247581852804817,0.0819282032302855));
#107874=CARTESIAN_POINT('',(-0.0321262178069016,-0.00552418147197183,0.0859282032302855));
#107875=CARTESIAN_POINT('Origin',(0.0161247821931084,0.00247581852803818,
0.0819282032302755));
#107876=CARTESIAN_POINT('Origin',(0.0161247821931084,-0.00552418147196183,
0.0859282032302755));
#107897=UNCERTAINTY_MEASURE_WITH_UNIT(LENGTH_MEASURE(1.E-5),#107911,
'DISTANCE_ACCURACY_VALUE',
'Maximum model space distance between geometric entities at asserted c
onnectivities');
#107898=UNCERTAINTY_MEASURE_WITH_UNIT(LENGTH_MEASURE(1.E-5),#107911,
'DISTANCE_ACCURACY_VALUE',
'Maximum model space distance between geometric entities at asserted c
onnectivities');
#107909=(
GEOMETRIC_REPRESENTATION_CONTEXT(3)
GLOBAL_UNCERTAINTY_ASSIGNED_CONTEXT((#107897))
GLOBAL_UNIT_ASSIGNED_CONTEXT((#107911,#107912,#107913))
REPRESENTATION_CONTEXT('','3D')
);
#107910=(
GEOMETRIC_REPRESENTATION_CONTEXT(3)
GLOBAL_UNCERTAINTY_ASSIGNED_CONTEXT((#107898))
GLOBAL_UNIT_ASSIGNED_CONTEXT((#107911,#107912,#107913))
REPRESENTATION_CONTEXT('','3D')
);
#107911=(
LENGTH_UNIT()
NAMED_UNIT(*)
SI_UNIT($,.METRE.)
);
#107912=(
NAMED_UNIT(*)
PLANE_ANGLE_UNIT()
SI_UNIT($,.RADIAN.)
);
#107913=(
NAMED_UNIT(*)
SI_UNIT($,.STERADIAN.)
SOLID_ANGLE_UNIT()
);
#107924=SHAPE_DEFINITION_REPRESENTATION(#107935,#107956);
#107935=PRODUCT_DEFINITION_SHAPE('',$,#107968);
#107956=SHAPE_REPRESENTATION('',(#50173),#107909);
#107957=PRODUCT_DEFINITION_CONTEXT('part definition',#107992,'design');
#107968=PRODUCT_DEFINITION('Extruder Body','Extruder Body',#107979,#107957);
#107979=PRODUCT_DEFINITION_FORMATION('',$,#108004);
#107992=APPLICATION_CONTEXT('Managed model based 3d engineering');
#107993=PRODUCT_CONTEXT('part definition',#107992,'mechanical');
#108004=PRODUCT('Extruder Body','Extruder Body',
'LEGAL AND USAGE DISCLAIMER: this Data/Model is provided \X2\201C\X0\A
S IS\X2\201D\X0\ for informational and representational only. It is a 
geometric approximation and is NOT engineered, certified, or guarantee
d for dimensional accuracy, exact tolerances, or production-level prec
ision. Vendor disclaims all implied warranties including fitness for a
 particular purpose. DO NOT USE FOR DIRECT PHYSICAL MANUFACTURING, AUT
OMATED PRODUCTION, OR SAFETY-CRITICAL SYSTEMS without independent engi
neering verification and resolution of any design discrepancies.',(#107993));
#108007=PRESENTATION_STYLE_ASSIGNMENT((#108014));
#108014=SURFACE_STYLE_USAGE(.BOTH.,#108021);
#108021=SURFACE_SIDE_STYLE('',(#108028));
#108028=SURFACE_STYLE_FILL_AREA(#108035);
#108035=FILL_AREA_STYLE('Opaque(48,59,150)',(#108042));
#108042=FILL_AREA_STYLE_COLOUR('Opaque(48,59,150)',#108049);
#108049=COLOUR_RGB('Opaque(48,59,150)',0.188235294117647,0.231372549019608,
0.588235294117647);
ENDSEC;
END-ISO-10303-21;
